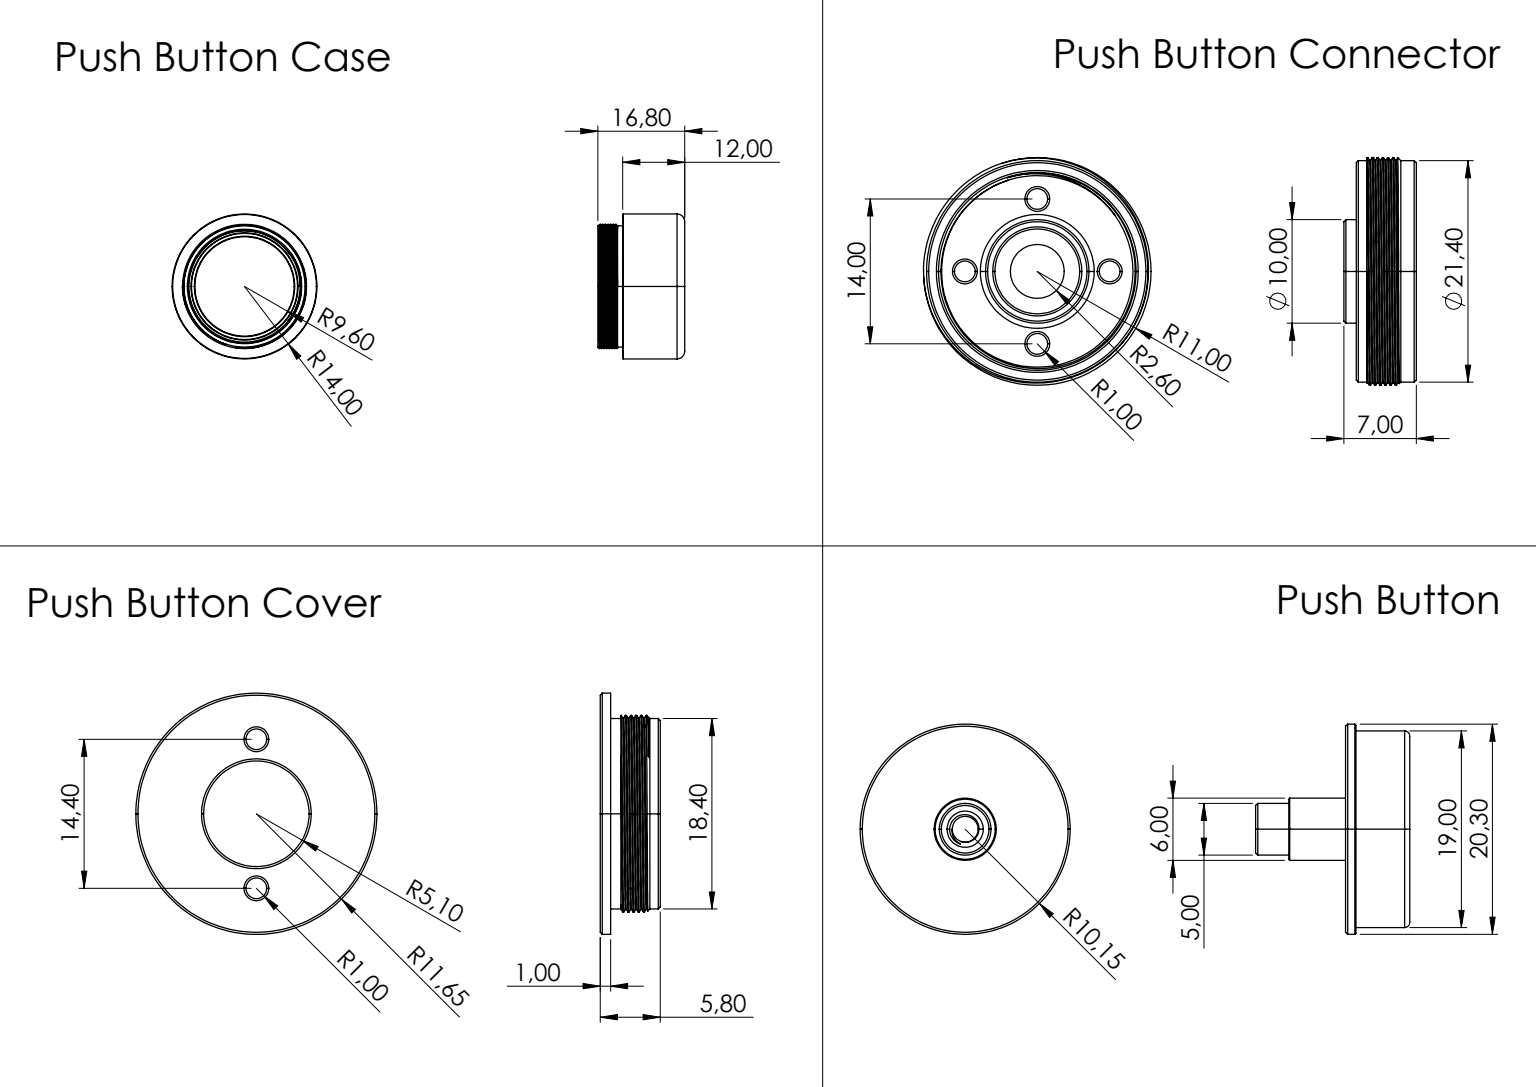
ISO-10303-21;
HEADER;
FILE_DESCRIPTION (('STEP AP214'),
    '1' );
FILE_NAME ('Push Button Cover.step',
    '2026-10-07T19:06:49',
    ( '' ),
    ( '' ),
    'SwSTEP 2.0',
    'SolidWorks 2020',
    '' );
FILE_SCHEMA (( 'AUTOMOTIVE_DESIGN' ));
ENDSEC;

DATA;
#2=CARTESIAN_POINT ( 'NONE',  ( 2.783482194004999855, -79.54451332859899537, 9.108908728793998932 ) ) ;
#10=ORIENTED_EDGE ( 'NONE', *, *, #20290, .T. ) ;
#20=CARTESIAN_POINT ( 'NONE',  ( 4.897371265365999982, -76.96065194988499059, 7.847181321287999722 ) ) ;
#42=CARTESIAN_POINT ( 'NONE',  ( -6.243826001791999758, -76.87571332859899087, 7.064314876436000645 ) ) ;
#56=CARTESIAN_POINT ( 'NONE',  ( 1.899930039692999895, -78.36919415034600434, 9.535935523283001203 ) ) ;
#70=FACE_OUTER_BOUND ( 'NONE', #58213, .T. ) ;
#83=AXIS2_PLACEMENT_3D ( 'NONE', #16611, #21316, #34596 ) ;
#85=CARTESIAN_POINT ( 'NONE',  ( -11.65000000000000036, -75.20000000000000284, 0.000000000000000000 ) ) ;
#89=VERTEX_POINT ( 'NONE', #22267 ) ;
#93=CARTESIAN_POINT ( 'NONE',  ( 3.039902587998999817, -77.28013998579800159, -9.045419714114000698 ) ) ;
#100=CARTESIAN_POINT ( 'NONE',  ( -9.706274203897999442, -78.20406332859900544, -1.344096209030999800 ) ) ;
#101=FACE_OUTER_BOUND ( 'NONE', #29091, .T. ) ;
#107=B_SPLINE_CURVE_WITH_KNOTS ( 'NONE', 3,
 ( #7548, #48867, #4281, #31114, #3130, #21981 ),
 .UNSPECIFIED., .F., .F.,
 ( 4, 2, 4 ),
 ( 0.000000000000000000, 0.5000000000000000000, 1.000000000000000000 ),
 .UNSPECIFIED. ) ;
#109=CARTESIAN_POINT ( 'NONE',  ( 1.243547092045969915, -77.53541666666666288, -9.500000000000000000 ) ) ;
#111=CARTESIAN_POINT ( 'NONE',  ( -5.219189444926520594, -79.47847823290939573, -7.938071756665344481 ) ) ;
#112=DIRECTION ( 'NONE',  ( 0.000000000000000000, 0.7071067811866525998, -0.7071067811864425456 ) ) ;
#113=CARTESIAN_POINT ( 'NONE',  ( -5.761654615528584600, -79.37404003602567570, -7.593432905074549488 ) ) ;
#124=CARTESIAN_POINT ( 'NONE',  ( 0.000000000000000000, -75.00000000000000000, -7.200000000000000178 ) ) ;
#131=CARTESIAN_POINT ( 'NONE',  ( 8.300970689365456678, -78.50833333333332575, -4.784380313523530326 ) ) ;
#138=CARTESIAN_POINT ( 'NONE',  ( 2.459440699436000077, -77.29584903538302854, -9.171074077620000153 ) ) ;
#141=CARTESIAN_POINT ( 'NONE',  ( -9.499999999999998224, -77.31041666666664014, -1.243547092045960367 ) ) ;
#182=CARTESIAN_POINT ( 'NONE',  ( -9.065329452404249366, -79.37552650030312407, 2.840436040226053560 ) ) ;
#198=AXIS2_PLACEMENT_3D ( 'NONE', #57985, #8985, #18719 ) ;
#217=CARTESIAN_POINT ( 'NONE',  ( 8.824144518603999288, -79.29006001420199823, -3.570895061352000077 ) ) ;
#227=FACE_OUTER_BOUND ( 'NONE', #43271, .T. ) ;
#233=VERTEX_POINT ( 'NONE', #25182 ) ;
#261=CARTESIAN_POINT ( 'NONE',  ( -7.282392150664000141, -77.69888667140099869, 6.502067388700999651 ) ) ;
#294=CARTESIAN_POINT ( 'NONE',  ( 8.002843206562666012, -78.09666666666663559, 5.305121725754472273 ) ) ;
#311=AXIS2_PLACEMENT_3D ( 'NONE', #35658, #30929, #8510 ) ;
#318=CARTESIAN_POINT ( 'NONE',  ( 7.430757984336000099, -77.37342305011499377, 5.911115298933000695 ) ) ;
#336=CARTESIAN_POINT ( 'NONE',  ( 8.828604248290998768, -77.09468998579799859, -4.107095029376999662 ) ) ;
#343=CARTESIAN_POINT ( 'NONE',  ( -9.500000000000000000, -77.79999999999999716, 0.000000000000000000 ) ) ;
#346=CARTESIAN_POINT ( 'NONE',  ( 8.913108430814103755, -77.00000000000000000, -3.200251741501357383 ) ) ;
#347=LINE ( 'NONE', #54049, #11944 ) ;
#348=CARTESIAN_POINT ( 'NONE',  ( 1.899930039692999895, -78.42929805011500832, 9.535935523283001203 ) ) ;
#359=DIRECTION ( 'NONE',  ( 0.000000000000000000, 1.000000000000000000, 0.000000000000000000 ) ) ;
#373=DIRECTION ( 'NONE',  ( 1.000000000000000000, 0.000000000000000000, 0.000000000000000000 ) ) ;
#376=( LENGTH_UNIT ( ) NAMED_UNIT ( * ) SI_UNIT ( .MILLI., .METRE. ) );
#389=CARTESIAN_POINT ( 'NONE',  ( -3.218338554480999925, -78.22738998579799841, -9.136931980783000284 ) ) ;
#395=EDGE_LOOP ( 'NONE', ( #41385, #43194, #13742, #37838 ) ) ;
#401=CARTESIAN_POINT ( 'NONE',  ( -8.419758540101616617, -79.43829028770473144, -4.400681399932081739 ) ) ;
#428=CARTESIAN_POINT ( 'NONE',  ( 0.7635722663974530144, -77.01859038055819440, 9.343284614800793975 ) ) ;
#503=CARTESIAN_POINT ( 'NONE',  ( -8.717770243732999802, -79.47198667140099815, 4.088898379276000306 ) ) ;
#504=DIRECTION ( 'NONE',  ( 0.000000000000000000, 1.000000000000000000, 0.000000000000000000 ) ) ;
#535=ORIENTED_EDGE ( 'NONE', *, *, #50020, .F. ) ;
#536=DIRECTION ( 'NONE',  ( 0.000000000000000000, 0.7071067811866525998, -0.7071067811864425456 ) ) ;
#549=CARTESIAN_POINT ( 'NONE',  ( -6.920864301812000186, -77.01268501420199186, 6.182201926393999791 ) ) ;
#601=ADVANCED_FACE ( 'NONE', ( #35967 ), #30933, .T. ) ;
#609=CARTESIAN_POINT ( 'NONE',  ( 8.256620083228000340, -77.33895194988498645, -4.688888258373000717 ) ) ;
#627=CARTESIAN_POINT ( 'NONE',  ( 9.014599915542000019, -77.66018998579799870, 3.680982378367999797 ) ) ;
#630=MECHANICAL_DESIGN_GEOMETRIC_PRESENTATION_REPRESENTATION('',(#12843),#25113);
#636=CARTESIAN_POINT ( 'NONE',  ( 9.443547551318811628, -77.00000000000000000, 0.1845321678459553028 ) ) ;
#643=CARTESIAN_POINT ( 'NONE',  ( 6.099999999940000528, -80.79999999975800051, 5.338249915816000005E-09 ) ) ;
#674=ORIENTED_EDGE ( 'NONE', *, *, #44519, .F. ) ;
#705=FACE_OUTER_BOUND ( 'NONE', #29095, .T. ) ;
#742=ORIENTED_EDGE ( 'NONE', *, *, #42939, .F. ) ;
#752=CARTESIAN_POINT ( 'NONE',  ( -3.329695900066999670, -78.41871001420200571, -9.453077866293002174 ) ) ;
#759=DIRECTION ( 'NONE',  ( 0.000000000000000000, 0.000000000000000000, -1.000000000000000000 ) ) ;
#773=CARTESIAN_POINT ( 'NONE',  ( -5.809342935555999787, -78.93238667140099096, 7.891128111295000025 ) ) ;
#806=CARTESIAN_POINT ( 'NONE',  ( 9.468750000004000356, -79.53124999999600675, -6.681056941828999630E-10 ) ) ;
#821=EDGE_CURVE ( 'NONE', #25723, #3607, #50108, .T. ) ;
#839=CARTESIAN_POINT ( 'NONE',  ( -8.920186055527000946, -77.16191332859899887, 3.688297430249000364 ) ) ;
#845=FACE_OUTER_BOUND ( 'NONE', #7013, .T. ) ;
#866=CARTESIAN_POINT ( 'NONE',  ( 0.9783655976132111798, -77.00000000000000000, 9.249733681752722703 ) ) ;
#869=CARTESIAN_POINT ( 'NONE',  ( 9.235752227612000098, -79.39493998579798983, 1.834089355993999915 ) ) ;
#887=EDGE_CURVE ( 'NONE', #29780, #37236, #38592, .T. ) ;
#892=CARTESIAN_POINT ( 'NONE',  ( 1.009320482739999969, -77.49657694988499657, 9.441330439200999791 ) ) ;
#901=CARTESIAN_POINT ( 'NONE',  ( -8.300970689365472666, -77.75833333333333997, 4.784380313523514339 ) ) ;
#956=CARTESIAN_POINT ( 'NONE',  ( 1.958352037450999727, -78.23868998579800405, 9.829161269560000136 ) ) ;
#1007=CARTESIAN_POINT ( 'NONE',  ( 7.056385154380720337, -79.75000000000000000, -6.024759004142000940 ) ) ;
#1024=CARTESIAN_POINT ( 'NONE',  ( 9.252740428349003565, -78.02916666666668277, -2.486604901413146607 ) ) ;
#1039=CARTESIAN_POINT ( 'NONE',  ( -0.5475862000146000108, -78.94131001420200278, -10.00738244094000073 ) ) ;
#1054=CARTESIAN_POINT ( 'NONE',  ( -9.221371799403371483, -77.06727193750342053, -2.052095926117649682 ) ) ;
#1057=CARTESIAN_POINT ( 'NONE',  ( -7.459109567305000077, -79.06303667140099378, -6.354485205484000865 ) ) ;
#1075=CARTESIAN_POINT ( 'NONE',  ( -8.895437731725001740, -79.41463998579799011, -4.226908468493999038 ) ) ;
#1091=AXIS2_PLACEMENT_3D ( 'NONE', #18206, #13750, #55665 ) ;
#1119=CARTESIAN_POINT ( 'NONE',  ( 9.515085579998999066, -77.75946167140099874, 0.3080020932329999850 ) ) ;
#1130=CARTESIAN_POINT ( 'NONE',  ( 6.100000000000000533, -80.79999999999999716, 0.000000000000000000 ) ) ;
#1134=EDGE_CURVE ( 'NONE', #37723, #31238, #6712, .T. ) ;
#1136=CARTESIAN_POINT ( 'NONE',  ( 4.009386773507102042, -79.41013248972129190, -8.520383303337226266 ) ) ;
#1158=CARTESIAN_POINT ( 'NONE',  ( 6.052764987364000149, -79.37291332859899740, -7.354162135516000731 ) ) ;
#1177=CARTESIAN_POINT ( 'NONE',  ( -9.204193785523999694, -77.14980194988498852, -2.332437886131999871 ) ) ;
#1204=CYLINDRICAL_SURFACE ( 'NONE', #30513, 9.500000000000000000 ) ;
#1213=CIRCLE ( 'NONE', #8729, 9.499999999999996447 ) ;
#1230=B_SPLINE_CURVE_WITH_KNOTS ( 'NONE', 3,
 ( #22828, #141, #18409, #57669, #53244, #53839, #17225, #26948, #36401, #54129, #35214, #44981, #40248, #35809, #35510, #13670, #31666, #12793 ),
 .UNSPECIFIED., .F., .F.,
 ( 4, 2, 2, 2, 2, 2, 2, 2, 4 ),
 ( 0.000000000000000000, 0.1250000000000000833, 0.2500000000000001665, 0.3750000000000002220, 0.5000000000000002220, 0.6250000000000002220, 0.7500000000000001110, 0.8750000000000001110, 1.000000000000000000 ),
 .UNSPECIFIED. ) ;
#1240=CARTESIAN_POINT ( 'NONE',  ( 6.874531804813999614, -78.06448998579800502, -7.293035489291000317 ) ) ;
#1246=CARTESIAN_POINT ( 'NONE',  ( -8.428125188755409170, -79.36138179854771124, 4.406741964346048590 ) ) ;
#1258=CARTESIAN_POINT ( 'NONE',  ( 9.500000000000000000, -79.14999999999999147, 0.000000000000000000 ) ) ;
#1283=CARTESIAN_POINT ( 'NONE',  ( 7.479653633103032995, -77.95140769025543648, 5.651087642253929566 ) ) ;
#1299=CARTESIAN_POINT ( 'NONE',  ( -1.000000000000000000, -78.00000000000000000, 7.200000000000000178 ) ) ;
#1304=CARTESIAN_POINT ( 'NONE',  ( 8.300970689365456678, -78.00833333333332575, -4.784380313523530326 ) ) ;
#1306=EDGE_CURVE ( 'NONE', #10320, #25686, #34712, .T. ) ;
#1317=VERTEX_POINT ( 'NONE', #7865 ) ;
#1326=ORIENTED_EDGE ( 'NONE', *, *, #45707, .F. ) ;
#1338=CARTESIAN_POINT ( 'NONE',  ( -8.932802644879007659, -77.57622193750340500, -3.074066805765899080 ) ) ;
#1366=CARTESIAN_POINT ( 'NONE',  ( 7.507056363060000237, -79.76904805011500343, -5.572808305725000189 ) ) ;
#1370=CARTESIAN_POINT ( 'NONE',  ( 9.252740428348992907, -77.17083333333333428, 2.486604901413179025 ) ) ;
#1386=ADVANCED_FACE ( 'NONE', ( #41198 ), #6893, .F. ) ;
#1416=CARTESIAN_POINT ( 'NONE',  ( -2.226051307435857662, -77.00624999999999432, -9.265603215652616242 ) ) ;
#1422=SHAPE_REPRESENTATION ( 'Push Button Cover', ( #43526 ), #24646 ) ;
#1426=CARTESIAN_POINT ( 'NONE',  ( -0.5312504855272001114, -78.63049415034599576, -9.708839960653000034 ) ) ;
#1499=EDGE_LOOP ( 'NONE', ( #5788, #41984, #28707, #17470, #27775, #26159 ) ) ;
#1517=CARTESIAN_POINT ( 'NONE',  ( -9.155305986995932344, -76.99999999999998579, 1.687095892431314637 ) ) ;
#1527=EDGE_CURVE ( 'NONE', #5139, #52771, #40497, .T. ) ;
#1531=CARTESIAN_POINT ( 'NONE',  ( -8.093517052318336624, -79.35576814611899010, 4.979337055998752426 ) ) ;
#1540=ORIENTED_EDGE ( 'NONE', *, *, #15656, .T. ) ;
#1568=CYLINDRICAL_SURFACE ( 'NONE', #18933, 1.000000000000000000 ) ;
#1581=AXIS2_PLACEMENT_3D ( 'NONE', #4302, #35280, #26150 ) ;
#1584=AXIS2_PLACEMENT_3D ( 'NONE', #55642, #9900, #14892 ) ;
#1608=CARTESIAN_POINT ( 'NONE',  ( 7.265173101945999967, -78.12837668086899612, 6.414655419558000560 ) ) ;
#1631=CARTESIAN_POINT ( 'NONE',  ( -9.595602112029999020, -78.08161001420199909, -1.328770664336999863 ) ) ;
#1639=CARTESIAN_POINT ( 'NONE',  ( 0.000000000000000000, -80.79999999999999716, -9.000000000000000000 ) ) ;
#1650=CARTESIAN_POINT ( 'NONE',  ( 1.848914204786999971, -79.30291332859900422, 9.561723555723999013 ) ) ;
#1652=CARTESIAN_POINT ( 'NONE',  ( 0.000000000000000000, -79.79999999999999716, -9.199999999999999289 ) ) ;
#1659=CARTESIAN_POINT ( 'NONE',  ( -6.090475762158000350, -79.49994805011499466, 7.362120511650999788 ) ) ;
#1679=CARTESIAN_POINT ( 'NONE',  ( 7.689480989199970473, -79.19964970209089472, 5.578385363880753012 ) ) ;
#1686=DIRECTION ( 'NONE',  ( 0.000000000000000000, 1.000000000000000000, 0.000000000000000000 ) ) ;
#1695=CARTESIAN_POINT ( 'NONE',  ( 8.533343070146999665, -77.28601001420200589, -3.969738581741999450 ) ) ;
#1700=CARTESIAN_POINT ( 'NONE',  ( 6.799660072434999591, -77.38031332859900147, -6.851122554325000280 ) ) ;
#1713=CARTESIAN_POINT ( 'NONE',  ( -3.039602602086000083, -79.10954415034599663, -9.236151215514999180 ) ) ;
#1738=ORIENTED_EDGE ( 'NONE', *, *, #53660, .F. ) ;
#1740=EDGE_CURVE ( 'NONE', #34146, #1317, #10335, .T. ) ;
#1746=ORIENTED_EDGE ( 'NONE', *, *, #40301, .T. ) ;
#1747=VERTEX_POINT ( 'NONE', #53544 ) ;
#1750=CARTESIAN_POINT ( 'NONE',  ( 8.582508435409000214, -76.84333998579799641, -4.171307237795000233 ) ) ;
#1762=CARTESIAN_POINT ( 'NONE',  ( 1.900228162289573586, -78.40847913613843900, 9.537431829883434631 ) ) ;
#1805=ADVANCED_BREP_SHAPE_REPRESENTATION ( '', ( #17895, #43526 ), #24646 ) ;
#1811=CARTESIAN_POINT ( 'NONE',  ( -7.401644128749154561, -77.00000000000002842, -5.852483073979606765 ) ) ;
#1825=AXIS2_PLACEMENT_3D ( 'NONE', #48424, #20395, #7104 ) ;
#1834=ORIENTED_EDGE ( 'NONE', *, *, #5380, .F. ) ;
#1858=CARTESIAN_POINT ( 'NONE',  ( -8.997179024602999675, -79.15920584965400053, 3.687079342327000298 ) ) ;
#1906=CARTESIAN_POINT ( 'NONE',  ( -5.674993058560000136, -78.89776001420199236, -8.260872093916999503 ) ) ;
#1911=VERTEX_POINT ( 'NONE', #57674 ) ;
#1918=CARTESIAN_POINT ( 'NONE',  ( 0.000000000000000000, -76.00000000000000000, 0.000000000000000000 ) ) ;
#1927=CARTESIAN_POINT ( 'NONE',  ( -0.5292728922702000238, -78.69131001420200278, -9.672698560386999489 ) ) ;
#1946=CARTESIAN_POINT ( 'NONE',  ( -6.239533324134999503, -79.44973998579799002, -7.619964241536999694 ) ) ;
#1952=CARTESIAN_POINT ( 'NONE',  ( 9.377128579935000374, -78.37869514476064126, -2.571625947824999869 ) ) ;
#1957=CARTESIAN_POINT ( 'NONE',  ( -2.317989000404999889, -79.73555194988499295, -9.269382932261999386 ) ) ;
#1968=B_SPLINE_CURVE_WITH_KNOTS ( 'NONE', 3,
 ( #13129, #31125, #31425, #49162, #26706, #40305, #58313, #17875, #23747, #14300, #10472, #28750, #1338, #41761, #15182, #28458, #46506, #6032, #46800, #32588, #5168, #41176, #10772, #24041, #32293, #28162, #33174, #36739, #37615, #55339, #1054, #27584, #5740, #54757, #42056 ),
 .UNSPECIFIED., .F., .F.,
 ( 4, 1, 1, 1, 1, 1, 1, 1, 1, 1, 1, 1, 1, 1, 1, 1, 1, 1, 1, 1, 1, 1, 1, 1, 1, 1, 1, 1, 1, 1, 1, 1, 4 ),
 ( 0.000000000000000000, 0.01250064086135114876, 0.04500059900521829331, 0.07750055714907158610, 0.1100005152929402902, 0.1425004734368089665, 0.1750004315807084654, 0.2075003897244847573, 0.2400003478684150648, 0.2725003060121913845, 0.3050002641561216365, 0.3375002223000519441, 0.3700001804438282638, 0.4025001385877585158, 0.4350000967315347800, 0.4675000548754650875, 0.5000000130192413517, 0.5324999711631716037, 0.5649999293071019668, 0.5974998874508783420, 0.6299998455948085940, 0.6624998037385848582, 0.6949997618825151102, 0.7274997200262914854, 0.7599996781702217374, 0.7924996363141521005, 0.8249995944579283647, 0.8574995526018586167, 0.8899995107456349919, 0.9224994688895652439, 0.9549994270333415081, 0.9874993851772717601, 1.000000000000000000 ),
 .UNSPECIFIED. ) ;
#1976=CARTESIAN_POINT ( 'NONE',  ( 8.331125690395985828, -79.18975047827684932, 4.575408606511675913 ) ) ;
#1991=ADVANCED_FACE ( 'NONE', ( #46760 ), #55002, .T. ) ;
#1992=DIRECTION ( 'NONE',  ( 0.000000000000000000, -1.000000000000000000, 0.000000000000000000 ) ) ;
#1998=CARTESIAN_POINT ( 'NONE',  ( 2.486604901413132840, -77.15416666666668277, 9.252740428349005342 ) ) ;
#2051=CARTESIAN_POINT ( 'NONE',  ( 9.426477049435000310, -77.25026915034599995, -1.139727483088999849 ) ) ;
#2055=CARTESIAN_POINT ( 'NONE',  ( -9.632966741362359642, -78.06007913613844096, -1.333944807945767863 ) ) ;
#2061=CARTESIAN_POINT ( 'NONE',  ( 1.243547092045969915, -78.03541666666666288, -9.500000000000000000 ) ) ;
#2065=CARTESIAN_POINT ( 'NONE',  ( -9.252740428349007118, -78.87916666666666288, 2.486604901413125734 ) ) ;
#2093=AXIS2_PLACEMENT_3D ( 'NONE', #49507, #50097, #22330 ) ;
#2109=CARTESIAN_POINT ( 'NONE',  ( -9.372585790538636275, -77.88499999999999091, 1.790612804732441221 ) ) ;
#2114=CARTESIAN_POINT ( 'NONE',  ( -9.379567534213441249, -79.38691803057906782, 1.514930929802611681 ) ) ;
#2146=FACE_OUTER_BOUND ( 'NONE', #52697, .T. ) ;
#2164=LINE ( 'NONE', #46757, #39820 ) ;
#2193=CARTESIAN_POINT ( 'NONE',  ( 6.711318802534000483, -78.57268667140098728, 7.292371261484999145 ) ) ;
#2212=CARTESIAN_POINT ( 'NONE',  ( 6.797895215277000247, -78.12826332859900447, -7.211733462747999646 ) ) ;
#2237=CARTESIAN_POINT ( 'NONE',  ( -8.918806285220000518, -78.11739514476064983, 3.872830773119999126 ) ) ;
#2246=CARTESIAN_POINT ( 'NONE',  ( 4.784380313523522332, -77.23333333333332007, 8.300970689365462007 ) ) ;
#2257=CARTESIAN_POINT ( 'NONE',  ( 6.135231488085603146, -79.21900635011196812, 7.253197741126338194 ) ) ;
#2278=CARTESIAN_POINT ( 'NONE',  ( -7.361960514518000487, -77.56153667140098662, -6.036001273387999966 ) ) ;
#2315=EDGE_LOOP ( 'NONE', ( #8172, #22576, #4098, #16468 ) ) ;
#2320=ORIENTED_EDGE ( 'NONE', *, *, #58012, .F. ) ;
#2324=ORIENTED_EDGE ( 'NONE', *, *, #52934, .F. ) ;
#2338=CARTESIAN_POINT ( 'NONE',  ( -5.506559303151407292, -78.62622913613842002, -8.015689466314336542 ) ) ;
#2346=CARTESIAN_POINT ( 'NONE',  ( -9.252740428349001789, -77.92083333333333428, -2.486604901413163926 ) ) ;
#2395=EDGE_LOOP ( 'NONE', ( #43208, #30951, #22703, #57067 ) ) ;
#2438=LINE ( 'NONE', #38724, #47230 ) ;
#2448=CARTESIAN_POINT ( 'NONE',  ( 4.044903269867999640, -79.05999999999998806, -8.595856998426999240 ) ) ;
#2475=CARTESIAN_POINT ( 'NONE',  ( 1.936520525790000002, -78.61623667140099769, 9.719586767747999900 ) ) ;
#2485=CARTESIAN_POINT ( 'NONE',  ( -9.450266643504305009, -79.40799665456589196, -0.9830318362740778637 ) ) ;
#2491=CARTESIAN_POINT ( 'NONE',  ( 8.546298008199000762, -78.65086332859900153, -5.018094164374000243 ) ) ;
#2494=CIRCLE ( 'NONE', #39213, 9.000000000000000000 ) ;
#2521=CARTESIAN_POINT ( 'NONE',  ( 8.384816012895999648, -78.85774514476065633, -4.923277454554000343 ) ) ;
#2542=CARTESIAN_POINT ( 'NONE',  ( 4.369668091130538556, -79.23660998577489067, 8.435227713305813779 ) ) ;
#2547=ORIENTED_EDGE ( 'NONE', *, *, #21590, .T. ) ;
#2550=CONICAL_SURFACE ( 'NONE', #34593, 9.099999999966000175, 0.7853981633972997312 ) ;
#2563=CARTESIAN_POINT ( 'NONE',  ( -5.838193839761721016, -77.22708333333332575, 7.596835002782687418 ) ) ;
#2578=VECTOR ( 'NONE', #112, 1000.000000000000000 ) ;
#2619=CARTESIAN_POINT ( 'NONE',  ( 3.861138328465000047, -76.85095248368000398, 8.493887087553000370 ) ) ;
#2624=CARTESIAN_POINT ( 'NONE',  ( -7.604857126344345630, -78.49557913613843141, 6.061321726079917482 ) ) ;
#2717=CARTESIAN_POINT ( 'NONE',  ( 4.411570631796044140, -76.99999999999998579, 8.157888388493256926 ) ) ;
#2721=CARTESIAN_POINT ( 'NONE',  ( 9.345760913908002010, -78.40230194988500045, 2.683384691900000174 ) ) ;
#2750=VERTEX_POINT ( 'NONE', #3102 ) ;
#2762=CARTESIAN_POINT ( 'NONE',  ( 4.349579488465999511, -79.03151332859899014, 8.780633650160998727 ) ) ;
#2779=CARTESIAN_POINT ( 'NONE',  ( 6.711318802534000483, -78.25891332859899308, 7.292371261484999145 ) ) ;
#2787=CARTESIAN_POINT ( 'NONE',  ( 3.938458446976999205, -79.30999999999998806, -8.369650235310999165 ) ) ;
#2809=CARTESIAN_POINT ( 'NONE',  ( 6.584508673715998128, -78.46579514476064787, 7.154582167228999090 ) ) ;
#2820=VERTEX_POINT ( 'NONE', #8379 ) ;
#2827=CARTESIAN_POINT ( 'NONE',  ( 8.035977331916674515, -79.19462052551928366, 5.075416816263699005 ) ) ;
#2833=CARTESIAN_POINT ( 'NONE',  ( 1.861192509982939169, -79.69030282387936381, -9.372352437101028499 ) ) ;
#2846=CARTESIAN_POINT ( 'NONE',  ( 7.412894021246999365, -77.70291167140099731, -5.973338413043999928 ) ) ;
#2852=CARTESIAN_POINT ( 'NONE',  ( 0.000000000000000000, -79.65000000003199432, 0.000000000000000000 ) ) ;
#2910=CARTESIAN_POINT ( 'NONE',  ( -9.003040227835604981, -79.32727112472369413, -3.132519729896531935 ) ) ;
#2916=CARTESIAN_POINT ( 'NONE',  ( -7.596835002782739821, -78.84791666666669130, 5.838193839761659731 ) ) ;
#2945=CARTESIAN_POINT ( 'NONE',  ( -3.012268937172999816, -79.85615333806700278, -9.005103130722002192 ) ) ;
#2968=CARTESIAN_POINT ( 'NONE',  ( 0.000000000000000000, -74.70999999999999375, 0.000000000000000000 ) ) ;
#3006=CARTESIAN_POINT ( 'NONE',  ( -7.530775182571000315, -78.18455194988499102, -6.150709233331999037 ) ) ;
#3012=VERTEX_POINT ( 'NONE', #46175 ) ;
#3014=DIRECTION ( 'NONE',  ( 0.000000000000000000, -1.000000000000000000, 0.000000000000000000 ) ) ;
#3038=EDGE_CURVE ( 'NONE', #22499, #1747, #34876, .T. ) ;
#3040=FILL_AREA_STYLE_COLOUR ( '', #28459 ) ;
#3047=EDGE_LOOP ( 'NONE', ( #11821, #26978, #6807, #19530, #9731, #11234 ) ) ;
#3051=CARTESIAN_POINT ( 'NONE',  ( -7.459109567305000077, -79.24926332859899958, -6.354485205484000865 ) ) ;
#3067=EDGE_CURVE ( 'NONE', #31891, #15380, #15330, .T. ) ;
#3070=CARTESIAN_POINT ( 'NONE',  ( -9.706274203897999442, -78.01783667140099965, -1.344096209030999800 ) ) ;
#3076=CARTESIAN_POINT ( 'NONE',  ( 4.784380313523556083, -78.96666666666669698, -8.300970689365444244 ) ) ;
#3094=CARTESIAN_POINT ( 'NONE',  ( 0.000000000000000000, -75.00000000000000000, 0.000000000000000000 ) ) ;
#3102=CARTESIAN_POINT ( 'NONE',  ( -11.65000000000000036, -76.00000000000000000, 0.000000000000000000 ) ) ;
#3124=CARTESIAN_POINT ( 'NONE',  ( -3.112989155534594321, -79.30136502081413141, 8.977538257521471721 ) ) ;
#3126=ORIENTED_EDGE ( 'NONE', *, *, #57860, .F. ) ;
#3130=CARTESIAN_POINT ( 'NONE',  ( 7.217860716171294655, -79.49333333333333940, -6.227832364471528770 ) ) ;
#3142=CARTESIAN_POINT ( 'NONE',  ( -9.001945887299001470, -77.53326167140099301, -3.097861235667999757 ) ) ;
#3205=CARTESIAN_POINT ( 'NONE',  ( -9.500350562740681681, -79.30722730559423894, -0.7959580027764865395 ) ) ;
#3206=CARTESIAN_POINT ( 'NONE',  ( 2.486604901413172808, -78.04583333333330586, -9.252740428348992907 ) ) ;
#3239=CARTESIAN_POINT ( 'NONE',  ( 5.875583596582999668, -79.57968667140100649, 7.634009735705999944 ) ) ;
#3259=CARTESIAN_POINT ( 'NONE',  ( -0.7479529023060000892, -77.80888084965400253, -9.465622776916999825 ) ) ;
#3289=LINE ( 'NONE', #43440, #55934 ) ;
#3295=CARTESIAN_POINT ( 'NONE',  ( -3.039602602086000083, -79.16964805011500061, -9.236151215514999180 ) ) ;
#3329=VECTOR ( 'NONE', #58150, 1000.000000000000114 ) ;
#3336=CARTESIAN_POINT ( 'NONE',  ( -7.675809325333999844, -78.31138667140099585, -6.269164879585000349 ) ) ;
#3387=CARTESIAN_POINT ( 'NONE',  ( 9.539544502573999551, -79.32444805011499511, 0.5400218831816999687 ) ) ;
#3394=CARTESIAN_POINT ( 'NONE',  ( 0.000000000000000000, -74.70999999999999375, 0.000000000000000000 ) ) ;
#3404=ORIENTED_EDGE ( 'NONE', *, *, #821, .T. ) ;
#3406=CARTESIAN_POINT ( 'NONE',  ( -1.469979871250949310, -79.28716761129145141, 9.385467292518239191 ) ) ;
#3454=CIRCLE ( 'NONE', #47809, 9.199999999999999289 ) ;
#3482=CARTESIAN_POINT ( 'NONE',  ( -7.898810015907999471, -77.87186001420199943, -5.922837236108999370 ) ) ;
#3507=EDGE_CURVE ( 'NONE', #40288, #25723, #28706, .T. ) ;
#3519=CARTESIAN_POINT ( 'NONE',  ( -5.199237357848000229, -79.90086001420199580, -8.238468209311999857 ) ) ;
#3538=CARTESIAN_POINT ( 'NONE',  ( 1.009320482739999969, -77.55668084965400055, 9.441330439200999791 ) ) ;
#3566=ORIENTED_EDGE ( 'NONE', *, *, #40614, .T. ) ;
#3571=CARTESIAN_POINT ( 'NONE',  ( 3.574993757284770979, -77.00000000000001421, 8.552566962383416183 ) ) ;
#3574=CARTESIAN_POINT ( 'NONE',  ( -5.764562846862999912, -78.99544805011498738, 7.830301022820999712 ) ) ;
#3606=CARTESIAN_POINT ( 'NONE',  ( -1.243547092045951263, -78.51458333333333428, -9.500000000000003553 ) ) ;
#3607=VERTEX_POINT ( 'NONE', #16531 ) ;
#3609=EDGE_LOOP ( 'NONE', ( #5179, #30253, #35549, #13398 ) ) ;
#3613=CARTESIAN_POINT ( 'NONE',  ( -9.565996717342001077, -79.14193998579798972, -1.527434585433000036 ) ) ;
#3618=ORIENTED_EDGE ( 'NONE', *, *, #47736, .F. ) ;
#3625=CARTESIAN_POINT ( 'NONE',  ( -6.673815826044733335, -79.46282625145217082, -6.760806027906673954 ) ) ;
#3641=CARTESIAN_POINT ( 'NONE',  ( -8.300970689365446020, -78.84166666666665435, -4.784380313523547201 ) ) ;
#3669=CARTESIAN_POINT ( 'NONE',  ( -2.317989000404999889, -79.61534415034599022, -9.269382932261999386 ) ) ;
#3687=CARTESIAN_POINT ( 'NONE',  ( 1.484863747559565628, -79.26247634984721913, 9.383218303840022756 ) ) ;
#3751=EDGE_CURVE ( 'NONE', #41331, #18799, #13852, .T. ) ;
#3768=CARTESIAN_POINT ( 'NONE',  ( 9.685708259213999582, -77.51688667140099653, 1.223589504196999966 ) ) ;
#3778=ADVANCED_FACE ( 'NONE', ( #29700 ), #29807, .T. ) ;
#3802=ADVANCED_FACE ( 'NONE', ( #42725 ), #11435, .T. ) ;
#3816=EDGE_CURVE ( 'NONE', #39245, #23213, #25284, .T. ) ;
#3824=CARTESIAN_POINT ( 'NONE',  ( 4.001451577097999923, -78.02955584965400249, 8.339717337904000161 ) ) ;
#3855=LINE ( 'NONE', #4444, #25802 ) ;
#3857=LINE ( 'NONE', #30990, #48551 ) ;
#3860=CARTESIAN_POINT ( 'NONE',  ( 6.584508673715999905, -78.50595584965400064, 7.154582167228999978 ) ) ;
#3866=CARTESIAN_POINT ( 'NONE',  ( 2.951189771924321192, -78.14999999999996305, 9.074256859245705797 ) ) ;
#3875=DIRECTION ( 'NONE',  ( 0.000000000000000000, -1.000000000000000000, 0.000000000000000000 ) ) ;
#3876=ORIENTED_EDGE ( 'NONE', *, *, #16713, .F. ) ;
#3896=CARTESIAN_POINT ( 'NONE',  ( 4.299985066278999568, -78.96773998579799070, 8.680515821880000260 ) ) ;
#3906=CARTESIAN_POINT ( 'NONE',  ( -9.500000000000001776, -77.41041666666667709, -1.243547092045959923 ) ) ;
#3915=CARTESIAN_POINT ( 'NONE',  ( -4.760969735703844741, -79.21703514507530031, 8.244157308523952565 ) ) ;
#3957=EDGE_CURVE ( 'NONE', #34611, #40996, #52472, .T. ) ;
#3973=CARTESIAN_POINT ( 'NONE',  ( -7.560040866215333111, -79.34781027512715923, 5.752875731716930119 ) ) ;
#4004=CARTESIAN_POINT ( 'NONE',  ( -7.941500096889264171, -78.94666666666665833, -5.274086223140034058 ) ) ;
#4023=ORIENTED_EDGE ( 'NONE', *, *, #56145, .T. ) ;
#4054=CARTESIAN_POINT ( 'NONE',  ( 6.922694868096999521, -76.94662000473400099, -6.559930598350000253 ) ) ;
#4061=CARTESIAN_POINT ( 'NONE',  ( -3.948661938011531092, -79.74013365314458213, -8.441925471967053340 ) ) ;
#4082=FACE_BOUND ( 'NONE', #6449, .T. ) ;
#4098=ORIENTED_EDGE ( 'NONE', *, *, #31074, .F. ) ;
#4108=ORIENTED_EDGE ( 'NONE', *, *, #3507, .T. ) ;
#4115=CARTESIAN_POINT ( 'NONE',  ( -7.264520526674999701, -77.74583084965399848, -6.114261184555999762 ) ) ;
#4140=CARTESIAN_POINT ( 'NONE',  ( -9.504662724600999368, -76.89676498579798647, -2.115138623684999608 ) ) ;
#4153=CARTESIAN_POINT ( 'NONE',  ( -5.600962501326000265, -77.99379805011500366, 7.948110234177999445 ) ) ;
#4160=CARTESIAN_POINT ( 'NONE',  ( -8.872994237323279521, -78.27000000000003865, 3.510218210012939100 ) ) ;
#4186=( NAMED_UNIT ( * ) SI_UNIT ( $, .STERADIAN. ) SOLID_ANGLE_UNIT ( ) );
#4190=CARTESIAN_POINT ( 'NONE',  ( -5.838193839761687265, -78.47291666666666288, -7.596835002782715840 ) ) ;
#4191=CARTESIAN_POINT ( 'NONE',  ( 0.6948940501455999064, -77.49853998579800418, 9.517234252032999109 ) ) ;
#4198=CARTESIAN_POINT ( 'NONE',  ( 7.022198843594999573, -77.93705665246400827, 6.200125618097000135 ) ) ;
#4211=CARTESIAN_POINT ( 'NONE',  ( -9.148289698020947824, -79.42135170196439731, -2.562996480311285019 ) ) ;
#4212=CARTESIAN_POINT ( 'NONE',  ( -9.500000000000000000, -74.70999999999999375, 0.000000000000000000 ) ) ;
#4238=CARTESIAN_POINT ( 'NONE',  ( 5.948947503763784894, -77.81911908264200406, 7.191054624583967048 ) ) ;
#4241=B_SPLINE_SURFACE_WITH_KNOTS ( 'NONE', 3, 3, ( 
 ( #33205, #51543, #46831, #24665, #45951, #46244, #6063, #20239, #14626, #42673, #28785, #37651, #15214, #6357, #24374, #19649, #42386, #32618, #11100 ),
 ( #55961, #10212, #15512, #23488, #1957, #37355, #19950, #41501, #50670, #29080, #38232, #56253, #47125, #15803, #50376, #9923, #41794, #28191, #23779 ),
 ( #27905, #1366, #46541, #5482, #14916, #19362, #55371, #32911, #50955, #1659, #10507, #28490, #24073, #42090, #3387, #42967, #39395, #7811, #16677 ),
 ( #52975, #34658, #25812, #34080, #3669, #21669, #43840, #21382, #33792, #7232, #57403, #38524, #48275, #16961, #34943, #29651, #29365, #30522, #20526 ) ),
 .UNSPECIFIED., .F., .F., .F.,
 ( 4, 4 ),
 ( 4, 1, 1, 1, 1, 1, 1, 1, 1, 1, 1, 1, 1, 1, 1, 1, 4 ),
 ( -0.4015584965371999937, 1.401558496537000043 ),
 ( 0.5889552238806000650, 0.6151492537313000275, 0.6413432835821000211, 0.6675373134327999836, 0.6937313432835999771, 0.7199253731343000506, 0.7461194029851000442, 0.7723134328358000067, 0.7985074626866000003, 0.8247014925372999627, 0.8508955223880999563, 0.8770895522388000298, 0.9032835820896000234, 0.9294776119402999859, 0.9556716417910000594, 0.9818656716417999419, 1.008059701493000171 ),
 .UNSPECIFIED. ) ;
#4275=CARTESIAN_POINT ( 'NONE',  ( -5.548822036515788980, -79.32452569715752588, 7.710984173510062156 ) ) ;
#4281=CARTESIAN_POINT ( 'NONE',  ( 5.442299421053111708, -79.47333333333332916, -7.827182525635441479 ) ) ;
#4302=CARTESIAN_POINT ( 'NONE',  ( 0.000000000000000000, -75.20000000000000284, 0.000000000000000000 ) ) ;
#4305=CARTESIAN_POINT ( 'NONE',  ( -6.380391360217929630, -78.96666666666666856, -7.083361869089003449 ) ) ;
#4309=VERTEX_POINT ( 'NONE', #52100 ) ;
#4347=CARTESIAN_POINT ( 'NONE',  ( -8.160216722324735272, -79.66145833332932114, 4.702279492088285551 ) ) ;
#4356=CARTESIAN_POINT ( 'NONE',  ( -6.446975197297999394, -77.18928667140100686, 7.331209084132000342 ) ) ;
#4360=B_SPLINE_CURVE_WITH_KNOTS ( 'NONE', 3,
 ( #51971, #20663, #23923, #47560, #11528, #7085 ),
 .UNSPECIFIED., .F., .F.,
 ( 4, 2, 4 ),
 ( 0.000000000000000000, 0.5000000000000000000, 1.000000000000000000 ),
 .UNSPECIFIED. ) ;
#4365=CARTESIAN_POINT ( 'NONE',  ( -2.364557222828000072, -79.54490095943376105, 9.257622954664000758 ) ) ;
#4395=CARTESIAN_POINT ( 'NONE',  ( -2.978309893851999846, -79.79237999526598912, -8.903583414616999647 ) ) ;
#4413=CARTESIAN_POINT ( 'NONE',  ( 4.574312611392000072, -77.52515584965399853, 8.320643751074999983 ) ) ;
#4435=CARTESIAN_POINT ( 'NONE',  ( -8.084017119143000585, -76.98881332859899373, -5.230585977929000485 ) ) ;
#4444=CARTESIAN_POINT ( 'NONE',  ( -6.099999999940000528, -80.79999999975800051, -5.338250164827000611E-09 ) ) ;
#4445=CARTESIAN_POINT ( 'NONE',  ( 8.185698792048100358, -77.00000000000001421, 4.534146512987735633 ) ) ;
#4448=CARTESIAN_POINT ( 'NONE',  ( 6.584508673715999905, -78.38574805011499791, 7.154582167228999978 ) ) ;
#4455=CARTESIAN_POINT ( 'NONE',  ( -3.234762833941021931, -78.20250000000001478, 8.977080150340221110 ) ) ;
#4488=CARTESIAN_POINT ( 'NONE',  ( 9.022242495772999860, -77.35293998579798824, -3.108016392540000172 ) ) ;
#4496=CARTESIAN_POINT ( 'NONE',  ( 2.006136628026000235, -78.27093998579799461, -9.477164255927000625 ) ) ;
#4499=CARTESIAN_POINT ( 'NONE',  ( 4.790152371929814912, -79.21780269203372882, -7.968054111795736638 ) ) ;
#4506=CARTESIAN_POINT ( 'NONE',  ( -6.849002874435582200, -79.46067733726329152, -6.583439657378555410 ) ) ;
#4508=CARTESIAN_POINT ( 'NONE',  ( -0.6023433875411666749, -79.42080894732758622, -9.578712713088513908 ) ) ;
#4526=CARTESIAN_POINT ( 'NONE',  ( -8.300970689365446020, -78.34166666666668277, -4.784380313523547201 ) ) ;
#4533=CARTESIAN_POINT ( 'NONE',  ( 9.136202122873999798, -77.42194903538302242, 2.585973524421999237 ) ) ;
#4567=LINE ( 'NONE', #26395, #28221 ) ;
#4573=CARTESIAN_POINT ( 'NONE',  ( -7.688125331226709491, -79.34962435731765140, 5.580139227232765009 ) ) ;
#4592=CARTESIAN_POINT ( 'NONE',  ( -2.684723000728000297, -77.10913667140100358, -9.133676008435999805 ) ) ;
#4611=CARTESIAN_POINT ( 'NONE',  ( 9.504033308897000154, -79.32516001420199814, 0.5380116381770999601 ) ) ;
#4617=CARTESIAN_POINT ( 'NONE',  ( 3.350444873057258022, -79.30441504825350307, -8.644740048361368778 ) ) ;
#4661=CARTESIAN_POINT ( 'NONE',  ( -5.497893974011999418, -77.39866001420199382, -8.200266008636999615 ) ) ;
#4668=CARTESIAN_POINT ( 'NONE',  ( -6.188001695094492050, -79.71856730628915955, -7.220675648484128573 ) ) ;
#4685=PLANE ( 'NONE',  #14153 ) ;
#4696=CARTESIAN_POINT ( 'NONE',  ( -5.083316206963999662, -79.77331332859898794, -8.054784978366999582 ) ) ;
#4715=CARTESIAN_POINT ( 'NONE',  ( 9.475051992780000987, -77.81477305011499368, -0.6170397550469999270 ) ) ;
#4732=DIRECTION ( 'NONE',  ( 0.000000000000000000, 1.000000000000000000, 0.000000000000000000 ) ) ;
#4734=CARTESIAN_POINT ( 'NONE',  ( -4.454645851891000596, -77.35638832859899594, 8.536186251725998986 ) ) ;
#4742=CARTESIAN_POINT ( 'NONE',  ( 8.534835205664490942, -77.00000000000000000, 3.862497297122138296 ) ) ;
#4776=CARTESIAN_POINT ( 'NONE',  ( -2.486604901413153268, -78.50416666666667709, -9.252740428348998236 ) ) ;
#4784=CARTESIAN_POINT ( 'NONE',  ( 9.685875573750999834, -78.88063998579799829, 0.1582452683012000039 ) ) ;
#4799=CARTESIAN_POINT ( 'NONE',  ( -9.380299113924060350, -79.41227555779782676, -1.501938252706041643 ) ) ;
#4801=CARTESIAN_POINT ( 'NONE',  ( 0.000000000000000000, -77.00000000000000000, 0.000000000000000000 ) ) ;
#4815=PRODUCT_DEFINITION ( 'UNKNOWN', '', #22577, #7968 ) ;
#4825=CARTESIAN_POINT ( 'NONE',  ( 7.430757984335999211, -77.45347403538301023, 5.911115298933000695 ) ) ;
#4852=CARTESIAN_POINT ( 'NONE',  ( -5.100000000000000533, -76.79999999999999716, 0.000000000000000000 ) ) ;
#4859=CIRCLE ( 'NONE', #35929, 1.000000000000000000 ) ;
#4943=CARTESIAN_POINT ( 'NONE',  ( -1.179576631548999943, -77.45566001420199598, 9.337310497832001843 ) ) ;
#4964=ORIENTED_EDGE ( 'NONE', *, *, #37684, .T. ) ;
#4980=CARTESIAN_POINT ( 'NONE',  ( -3.858678039026999684, -79.53793998579800473, 8.589155328362998887 ) ) ;
#5002=CARTESIAN_POINT ( 'NONE',  ( 2.459440699436000077, -77.21579805011499786, -9.171074077620000153 ) ) ;
#5003=FACE_OUTER_BOUND ( 'NONE', #38346, .T. ) ;
#5013=CONICAL_SURFACE ( 'NONE', #36113, 1.099999997157999232, 0.7853981633972997312 ) ;
#5020=CARTESIAN_POINT ( 'NONE',  ( 4.982928723802999116, -77.54708998579799584, -8.365578579050000130 ) ) ;
#5032=CARTESIAN_POINT ( 'NONE',  ( -8.997179024602999675, -78.97889415034599381, 3.687079342327000298 ) ) ;
#5056=B_SPLINE_CURVE_WITH_KNOTS ( 'NONE', 3,
 ( #28202, #35965, #22688, #294, #54287, #31823 ),
 .UNSPECIFIED., .F., .F.,
 ( 4, 2, 4 ),
 ( 0.000000000000000000, 0.4999999999999998890, 1.000000000000000000 ),
 .UNSPECIFIED. ) ;
#5060=CARTESIAN_POINT ( 'NONE',  ( -8.314650709467036549, -77.00000000000000000, -4.397163425340465892 ) ) ;
#5116=CIRCLE ( 'NONE', #39063, 9.000000000000000000 ) ;
#5118=CARTESIAN_POINT ( 'NONE',  ( -2.205007487985999770, -77.04364903538302656, 9.235565851336001941 ) ) ;
#5139=VERTEX_POINT ( 'NONE', #49750 ) ;
#5168=CARTESIAN_POINT ( 'NONE',  ( 7.630512808711405803, -77.35002193750341348, 5.569571266600500614 ) ) ;
#5172=CARTESIAN_POINT ( 'NONE',  ( 7.890654042133999901, -77.86386001420198966, 4.760698198672999482 ) ) ;
#5179=ORIENTED_EDGE ( 'NONE', *, *, #6097, .F. ) ;
#5209=DIRECTION ( 'NONE',  ( 0.000000000000000000, -1.000000000000000000, 0.000000000000000000 ) ) ;
#5213=ORIENTED_EDGE ( 'NONE', *, *, #56640, .F. ) ;
#5219=CARTESIAN_POINT ( 'NONE',  ( 9.319018100775748437, -79.16524970259979455, 1.846458293751403135 ) ) ;
#5234=CARTESIAN_POINT ( 'NONE',  ( 8.924962326551000302, -77.79496001420199036, -2.986943611218999983 ) ) ;
#5239=CARTESIAN_POINT ( 'NONE',  ( -9.632028597164000061, -77.19831332859899931, -0.6303035207593999933 ) ) ;
#5268=CARTESIAN_POINT ( 'NONE',  ( -3.778637972659712574, -77.00000000000000000, 8.499186437672962668 ) ) ;
#5280=EDGE_LOOP ( 'NONE', ( #16907, #43622, #39884 ) ) ;
#5285=ORIENTED_EDGE ( 'NONE', *, *, #47801, .F. ) ;
#5290=CARTESIAN_POINT ( 'NONE',  ( -9.391369684923001060, -77.11827694988500070, 1.399863080762999923 ) ) ;
#5321=CARTESIAN_POINT ( 'NONE',  ( 7.685661446562000343, -77.00000000000000000, -5.583959896779000509 ) ) ;
#5332=CARTESIAN_POINT ( 'NONE',  ( 0.000000000000000000, -80.59999999999999432, 0.000000000000000000 ) ) ;
#5344=CARTESIAN_POINT ( 'NONE',  ( -8.944216015804251185, -77.00000000000000000, -2.811381416889873197 ) ) ;
#5351=CARTESIAN_POINT ( 'NONE',  ( -9.307291666739137881, -79.69270833332970483, -0.9752027189503162941 ) ) ;
#5355=CARTESIAN_POINT ( 'NONE',  ( -5.610847844242282001, -77.82499999999998863, 7.718163323371708628 ) ) ;
#5380=EDGE_CURVE ( 'NONE', #36499, #34323, #14580, .T. ) ;
#5406=CARTESIAN_POINT ( 'NONE',  ( 6.559824298179475655, -79.75000000000000000, -6.561935513396097264 ) ) ;
#5433=CARTESIAN_POINT ( 'NONE',  ( -0.8742025125545000996, -79.20261001420199420, 9.984153739810000872 ) ) ;
#5458=CARTESIAN_POINT ( 'NONE',  ( 8.449950666592000559, -78.71463667140099574, -4.961522297560000183 ) ) ;
#5473=CARTESIAN_POINT ( 'NONE',  ( 5.818877114584999788, -79.20403998579800486, 7.945831408065000545 ) ) ;
#5482=CARTESIAN_POINT ( 'NONE',  ( 1.861092857305999937, -79.71054805011500832, -9.371850619045000386 ) ) ;
#5517=ADVANCED_FACE ( 'NONE', ( #52071 ), #43580, .T. ) ;
#5521=CARTESIAN_POINT ( 'NONE',  ( 9.576515689347999682, -77.45311332859900233, 1.209795274715000257 ) ) ;
#5524=CARTESIAN_POINT ( 'NONE',  ( 9.500000000000005329, -77.14374999999998295, -0.7461282552275557700 ) ) ;
#5549=EDGE_LOOP ( 'NONE', ( #7465, #28790, #49499, #535, #12184, #37449, #17548, #17218, #35107 ) ) ;
#5553=CARTESIAN_POINT ( 'NONE',  ( 4.024324870012000233, -79.29007331913099677, -8.363631784355000320 ) ) ;
#5573=CARTESIAN_POINT ( 'NONE',  ( -7.591316436381999821, -77.18132694988500475, -5.703451837412999659 ) ) ;
#5574=PLANE ( 'NONE',  #42337 ) ;
#5638=CARTESIAN_POINT ( 'NONE',  ( -2.370458031814262068, -77.79499999999998749, 9.242975026304343089 ) ) ;
#5665=CARTESIAN_POINT ( 'NONE',  ( 9.500517569907307447, -79.06045223105810749, 1.242907163946308069 ) ) ;
#5685=CARTESIAN_POINT ( 'NONE',  ( 9.426477049435000310, -77.39042403538302040, -1.139727483088999849 ) ) ;
#5705=CARTESIAN_POINT ( 'NONE',  ( 2.486604901413172364, -77.94583333333333997, -9.252740428348998236 ) ) ;
#5740=CARTESIAN_POINT ( 'NONE',  ( -8.539484132404522754, -77.01652175453601501, 3.808411293863636971 ) ) ;
#5776=CARTESIAN_POINT ( 'NONE',  ( -5.838193839761721016, -77.32708333333333428, 7.596835002782687418 ) ) ;
#5787=ORIENTED_EDGE ( 'NONE', *, *, #54972, .T. ) ;
#5788=ORIENTED_EDGE ( 'NONE', *, *, #29018, .F. ) ;
#5797=DIRECTION ( 'NONE',  ( -1.000000000000000000, 0.000000000000000000, 0.000000000000000000 ) ) ;
#5807=CARTESIAN_POINT ( 'NONE',  ( -4.354206273205999622, -77.48393501420198959, 8.343719559825000687 ) ) ;
#5808=CARTESIAN_POINT ( 'NONE',  ( 0.000000000000000000, -79.65000000003199432, 0.000000000000000000 ) ) ;
#5813=VECTOR ( 'NONE', #19084, 1000.000000000000000 ) ;
#5814=CARTESIAN_POINT ( 'NONE',  ( 4.153738564337000838, -77.85351332859899287, -8.713191203520999295 ) ) ;
#5843=CARTESIAN_POINT ( 'NONE',  ( -7.483407197968000801, -77.00000000000000000, 5.437013583706000297 ) ) ;
#5875=VERTEX_POINT ( 'NONE', #46209 ) ;
#5892=DIRECTION ( 'NONE',  ( 0.000000000000000000, 0.7071067811866525998, -0.7071067811864425456 ) ) ;
#5911=ORIENTED_EDGE ( 'NONE', *, *, #32682, .F. ) ;
#5922=CARTESIAN_POINT ( 'NONE',  ( -9.340210362350283901, -76.99999999999998579, 0.02720789100463689644 ) ) ;
#5932=CARTESIAN_POINT ( 'NONE',  ( -0.6017968039497372246, -77.78000000000000114, 9.523103445003338052 ) ) ;
#5937=CARTESIAN_POINT ( 'NONE',  ( -8.997332162609597006, -79.37373539064718386, 3.050007033374654508 ) ) ;
#5960=CARTESIAN_POINT ( 'NONE',  ( 8.538006731470160204, -79.08654938339437024, 4.209831911330708110 ) ) ;
#6016=CARTESIAN_POINT ( 'NONE',  ( -5.773189589619000195, -78.24451001420199248, 8.192511063987998554 ) ) ;
#6032=CARTESIAN_POINT ( 'NONE',  ( -1.184016694733479591, -77.43484693750340853, 9.372457216979636740 ) ) ;
#6035=CARTESIAN_POINT ( 'NONE',  ( 9.342221983604002133, -78.29936001420199432, -2.562053005734000077 ) ) ;
#6054=CARTESIAN_POINT ( 'NONE',  ( 4.145750262472000180, -79.10401332859899526, -8.580453259755000062 ) ) ;
#6059=CARTESIAN_POINT ( 'NONE',  ( -8.997179024602999675, -79.11904514476064776, 3.687079342326999853 ) ) ;
#6063=CARTESIAN_POINT ( 'NONE',  ( -8.630067035710000667, -79.72545584965399712, -4.100810385846999750 ) ) ;
#6069=CARTESIAN_POINT ( 'NONE',  ( 1.243547092045927949, -77.26458333333334849, 9.500000000000003553 ) ) ;
#6070=DIRECTION ( 'NONE',  ( 1.000000000000000000, 0.000000000000000000, 0.000000000000000000 ) ) ;
#6097=EDGE_CURVE ( 'NONE', #9880, #16336, #56791, .T. ) ;
#6098=FACE_BOUND ( 'NONE', #10057, .T. ) ;
#6104=DIRECTION ( 'NONE',  ( 0.000000000000000000, 1.000000000000000000, 0.000000000000000000 ) ) ;
#6121=CARTESIAN_POINT ( 'NONE',  ( -3.339615680726000235, -78.47284805011499031, 9.131854552393999569 ) ) ;
#6137=CARTESIAN_POINT ( 'NONE',  ( -6.722422115750747551, -77.00000000000001421, 6.387398339048315776 ) ) ;
#6164=CARTESIAN_POINT ( 'NONE',  ( 4.897371265365999982, -76.84044415034598785, 7.847181321287999722 ) ) ;
#6182=EDGE_CURVE ( 'NONE', #6658, #11325, #42218, .T. ) ;
#6204=EDGE_LOOP ( 'NONE', ( #41155, #40324, #6266, #38099 ) ) ;
#6223=CARTESIAN_POINT ( 'NONE',  ( -0.8742025125545000996, -78.76128998579800111, 9.984153739810000872 ) ) ;
#6228=CARTESIAN_POINT ( 'NONE',  ( -9.034604909256527705, -79.37471052910895253, 2.936440201109655312 ) ) ;
#6239=DIRECTION ( 'NONE',  ( 0.000000000000000000, 1.000000000000000000, -4.899618830983999950E-14 ) ) ;
#6248=CARTESIAN_POINT ( 'NONE',  ( 7.156381309732353202, -79.10742710526332644, 6.276394420187332734 ) ) ;
#6260=CARTESIAN_POINT ( 'NONE',  ( 6.482950081930999531, -79.37695584965399576, -6.598019266050999754 ) ) ;
#6266=ORIENTED_EDGE ( 'NONE', *, *, #1740, .F. ) ;
#6300=CARTESIAN_POINT ( 'NONE',  ( 6.002077433942410778, -78.07088160286059519, 7.255254208431503038 ) ) ;
#6331=CARTESIAN_POINT ( 'NONE',  ( -7.575359187103000380, -78.51711001420200375, 6.037810896484000267 ) ) ;
#6338=FACE_OUTER_BOUND ( 'NONE', #6898, .T. ) ;
#6349=CARTESIAN_POINT ( 'NONE',  ( 8.557689913033998508, -79.23271332859899019, 4.648766890461000223 ) ) ;
#6354=CARTESIAN_POINT ( 'NONE',  ( 1.899930039692999895, -78.50934514476064408, 9.535935523283001203 ) ) ;
#6357=CARTESIAN_POINT ( 'NONE',  ( 8.395992668097999712, -79.47975584965399776, 4.560928606276999808 ) ) ;
#6362=CARTESIAN_POINT ( 'NONE',  ( -2.486604901413195901, -77.29583333333334849, 9.252740428348989354 ) ) ;
#6373=ORIENTED_EDGE ( 'NONE', *, *, #35099, .T. ) ;
#6378=CARTESIAN_POINT ( 'NONE',  ( 7.552177422520572669, -79.20153084570749513, 5.764790892576884929 ) ) ;
#6388=DIRECTION ( 'NONE',  ( 1.000000000000000000, 0.000000000000000000, 0.000000000000000000 ) ) ;
#6446=CARTESIAN_POINT ( 'NONE',  ( 8.540261029602000065, -76.91613998579799727, 4.257270096473000365 ) ) ;
#6449=EDGE_LOOP ( 'NONE', ( #1746, #16754, #44944 ) ) ;
#6458=B_SPLINE_CURVE_WITH_KNOTS ( 'NONE', 3,
 ( #18405, #13960, #1283, #45865, #36688, #50000, #9546, #54424, #27529, #54703, #55281, #54991, #13666, #14540, #31662, #23407, #32533, #36978, #4825, #4533, #5685, #36396, #40834, #138, #27819, #54125, #27237, #18694, #41122, #26945, #45571, #5118, #428, #23114, #41417 ),
 .UNSPECIFIED., .F., .F.,
 ( 4, 1, 1, 1, 1, 1, 1, 1, 1, 1, 1, 1, 1, 1, 1, 1, 1, 1, 1, 1, 1, 1, 1, 1, 1, 1, 1, 1, 1, 1, 1, 1, 4 ),
 ( 0.000000000000000000, 0.01250096958943576128, 0.04500090495504436433, 0.07750084032066266448, 0.1100007756862671354, 0.1425007110518439757, 0.1750006464174760634, 0.2075005817831081512, 0.2400005171487402389, 0.2725004525143723266, 0.3050003878800044421, 0.3375003232454983904, 0.3700002586111305614, 0.4025001939767626213, 0.4350001293423947368, 0.4675000647080267968, 0.5000000000736588568, 0.5324999354391528605, 0.5649998708047848650, 0.5974998061704170915, 0.6299997415360490960, 0.6624996769016813225, 0.6949996122673132160, 0.7274995476329454425, 0.7599994829984393352, 0.7924994183640715617, 0.8249993537297034552, 0.8574992890953355706, 0.8899992244609679082, 0.9224991598265999126, 0.9549990951922320281, 0.9874990305577258098, 1.000000000000000000 ),
 .UNSPECIFIED. ) ;
#6459=CARTESIAN_POINT ( 'NONE',  ( -5.601841361836865651, -77.97297913613843434, 7.949357391288894625 ) ) ;
#6517=CARTESIAN_POINT ( 'NONE',  ( 8.163677614451000153, -77.67253998579799656, 4.925422544966999716 ) ) ;
#6546=DIRECTION ( 'NONE',  ( -1.044282756598000039E-09, -1.000000000000000000, 6.141137129051000072E-09 ) ) ;
#6557=CARTESIAN_POINT ( 'NONE',  ( 9.722066209057999231, -78.94145584965399109, 0.1588365413100999990 ) ) ;
#6602=CARTESIAN_POINT ( 'NONE',  ( 9.633138876124000660, -78.59291001420200473, 2.765897569310999948 ) ) ;
#6607=EDGE_LOOP ( 'NONE', ( #26105, #44296 ) ) ;
#6616=CARTESIAN_POINT ( 'NONE',  ( -1.937158916668030528, -79.75000000000000000, -9.096604487445336673 ) ) ;
#6622=CARTESIAN_POINT ( 'NONE',  ( 9.525749612248999298, -78.21536332859899687, 2.735063621234999687 ) ) ;
#6635=EDGE_CURVE ( 'NONE', #42830, #44850, #55599, .T. ) ;
#6644=CARTESIAN_POINT ( 'NONE',  ( 9.723265251863999481, -79.19761332859899028, 0.5504220888713000637 ) ) ;
#6658=VERTEX_POINT ( 'NONE', #21559 ) ;
#6673=CARTESIAN_POINT ( 'NONE',  ( 6.169502046027795394, -79.21861551698380310, 7.223965119394421208 ) ) ;
#6676=ORIENTED_EDGE ( 'NONE', *, *, #23431, .F. ) ;
#6694=FACE_OUTER_BOUND ( 'NONE', #20596, .T. ) ;
#6700=CARTESIAN_POINT ( 'NONE',  ( 11.65000000000000036, -76.00000000000000000, 0.000000000000000000 ) ) ;
#6706=CONICAL_SURFACE ( 'NONE', #27422, 1.099999997157999232, 0.7853981633972997312 ) ;
#6712=LINE ( 'NONE', #19420, #33954 ) ;
#6715=B_SPLINE_SURFACE_WITH_KNOTS ( 'NONE', 3, 3, ( 
 ( #34505, #38948, #3519, #12375, #39235, #48405, #29783, #7942, #17679, #25944, #35074, #43386, #12659, #35666, #12091, #47839, #21519, #7370, #30653 ),
 ( #25371, #2945, #56963, #39526, #17091, #52534, #30074, #53111, #25655, #48687, #43684, #3239, #21231, #23280, #49268, #36269, #27982, #14407, #53698 ),
 ( #49574, #4395, #4696, #41577, #54293, #31526, #22395, #23564, #13830, #10003, #2, #40406, #13235, #18856, #53995, #32406, #1158, #46030, #40998 ),
 ( #31229, #9121, #49870, #19146, #54583, #36561, #45736, #14123, #4980, #27693, #8821, #45438, #31828, #869, #50450, #32119, #50160, #5553, #9703 ) ),
 .UNSPECIFIED., .F., .F., .F.,
 ( 4, 4 ),
 ( 4, 1, 1, 1, 1, 1, 1, 1, 1, 1, 1, 1, 1, 1, 1, 1, 4 ),
 ( -0.1377334280162000046, 1.137733428016000081 ),
 ( 0.6650746268656999582, 0.6864179104477999838, 0.7077611940298000892, 0.7291044776119000037, 0.7504477611940000292, 0.7717910447760999437, 0.7931343283582000803, 0.8144776119402999948, 0.8358208955224000203, 0.8571641791044999348, 0.8785074626865999603, 0.8998507462686999858, 0.9211940298506999802, 0.9425373134328000058, 0.9638805970148999203, 0.9852238805970000568, 1.006567164178999940 ),
 .UNSPECIFIED. ) ;
#6748=CARTESIAN_POINT ( 'NONE',  ( 5.102724688570000389, -77.83873581701298860, 7.811319209985999379 ) ) ;
#6754=CARTESIAN_POINT ( 'NONE',  ( -8.920205756585657397, -78.01652913613843054, 3.873438468320558936 ) ) ;
#6807=ORIENTED_EDGE ( 'NONE', *, *, #15995, .F. ) ;
#6854=VECTOR ( 'NONE', #55885, 1000.000000000000000 ) ;
#6871=DIRECTION ( 'NONE',  ( 0.000000000000000000, 1.000000000000000000, 0.000000000000000000 ) ) ;
#6893=B_SPLINE_SURFACE_WITH_KNOTS ( 'NONE', 3, 3, ( 
 ( #48898, #53315, #45058, #12859, #54204, #8438, #40620, #36472, #22011, #40019, #9621, #31739, #58034, #14037, #4611, #217, #53610, #18193, #49783 ),
 ( #9330, #17594, #22307, #13149, #31143, #27320, #32032, #22901, #503, #49184, #50076, #27607, #8735, #26728, #44755, #58333, #17896, #35885, #19641 ),
 ( #23770, #46237, #19353, #9913, #41488, #33498, #46823, #51535, #29071, #28776, #41785, #1650, #50658, #6349, #6644, #32317, #37929, #6054, #19064 ),
 ( #24365, #24653, #10496, #27894, #42377, #1946, #1075, #37640, #42663, #11091, #37346, #45941, #5473, #19940, #18768, #55656, #14616, #14906, #55954 ) ),
 .UNSPECIFIED., .F., .F., .F.,
 ( 4, 4 ),
 ( 4, 1, 1, 1, 1, 1, 1, 1, 1, 1, 1, 1, 1, 1, 1, 1, 4 ),
 ( -0.1377334280162000046, 1.137733428016000081 ),
 ( 0.5889552238806000650, 0.6151492537313000275, 0.6413432835821000211, 0.6675373134327999836, 0.6937313432835999771, 0.7199253731343000506, 0.7461194029851000442, 0.7723134328358000067, 0.7985074626866000003, 0.8247014925372999627, 0.8508955223880999563, 0.8770895522388000298, 0.9032835820896000234, 0.9294776119402999859, 0.9556716417910000594, 0.9818656716417999419, 1.008059701493000171 ),
 .UNSPECIFIED. ) ;
#6895=CARTESIAN_POINT ( 'NONE',  ( -3.403932870613000095, -78.65978667140099390, 9.307723658127001087 ) ) ;
#6898=EDGE_LOOP ( 'NONE', ( #23795, #18909, #40759, #48072 ) ) ;
#6904=CARTESIAN_POINT ( 'NONE',  ( -9.500228589985420413, -79.40182418455218283, -0.2334504967788087748 ) ) ;
#6913=CARTESIAN_POINT ( 'NONE',  ( -5.875581754031000692, -78.86861332859899676, 7.981103691720999649 ) ) ;
#6941=CARTESIAN_POINT ( 'NONE',  ( -9.646692012709998210, -78.63999514476064689, 1.218660606027000215 ) ) ;
#6961=CARTESIAN_POINT ( 'NONE',  ( 9.052015793914058861, -79.17411443971855078, 2.882270040945727363 ) ) ;
#6963=FACE_OUTER_BOUND ( 'NONE', #39975, .T. ) ;
#6976=CARTESIAN_POINT ( 'NONE',  ( -1.983076715186758543, -79.52083333388351605, -9.322644982774999534 ) ) ;
#6982=CARTESIAN_POINT ( 'NONE',  ( 9.499999999999998224, -77.06041666666666856, 1.243547092045980129 ) ) ;
#7013=EDGE_LOOP ( 'NONE', ( #29303, #57828, #58365, #1834, #35011 ) ) ;
#7014=DIRECTION ( 'NONE',  ( 0.7071067811865474617, 0.7071067811865474617, -1.027168298793069202E-09 ) ) ;
#7038=CARTESIAN_POINT ( 'NONE',  ( 5.896171905175000560, -77.86999999999999034, 7.127247495676000355 ) ) ;
#7039=CARTESIAN_POINT ( 'NONE',  ( 6.214091009702999102, -77.69161915034599986, -7.179311535719000048 ) ) ;
#7052=CARTESIAN_POINT ( 'NONE',  ( -4.784380313523539208, -77.98333333333332007, -8.300970689365453126 ) ) ;
#7085=CARTESIAN_POINT ( 'NONE',  ( 9.468750000004000356, -79.53124999999600675, -6.681056941828999630E-10 ) ) ;
#7104=DIRECTION ( 'NONE',  ( -1.000000000000000000, 0.000000000000000000, 0.000000000000000000 ) ) ;
#7137=CARTESIAN_POINT ( 'NONE',  ( -5.600962501326000265, -78.11400584965400640, 7.948110234177999445 ) ) ;
#7183=CARTESIAN_POINT ( 'NONE',  ( -9.042797184480999562, -78.79043667140099672, -4.055650103703999143 ) ) ;
#7200=CARTESIAN_POINT ( 'NONE',  ( -9.721629130303000466, -78.49688667140098630, 1.228127365514999791 ) ) ;
#7223=CARTESIAN_POINT ( 'NONE',  ( 8.500869906239369556, -79.11249999999999716, -4.334382246026802221 ) ) ;
#7232=CARTESIAN_POINT ( 'NONE',  ( -6.090475762158000350, -79.43984415034599067, 7.362120511650999788 ) ) ;
#7251=CARTESIAN_POINT ( 'NONE',  ( 2.890496000096741014, -79.25013075116083883, 9.049465696841215490 ) ) ;
#7327=CARTESIAN_POINT ( 'NONE',  ( 8.386131694562763528, -78.75687913613843705, -4.924049977871809425 ) ) ;
#7370=CARTESIAN_POINT ( 'NONE',  ( 4.163570051248999704, -79.48139334753599883, -8.653020802693998093 ) ) ;
#7385=EDGE_CURVE ( 'NONE', #42268, #22499, #3289, .T. ) ;
#7397=ORIENTED_EDGE ( 'NONE', *, *, #42096, .T. ) ;
#7416=( NAMED_UNIT ( * ) SI_UNIT ( $, .STERADIAN. ) SOLID_ANGLE_UNIT ( ) );
#7427=CARTESIAN_POINT ( 'NONE',  ( -7.603664017118000551, -78.63660584965400346, 6.060370778711000384 ) ) ;
#7464=ORIENTED_EDGE ( 'NONE', *, *, #8298, .T. ) ;
#7465=ORIENTED_EDGE ( 'NONE', *, *, #18739, .F. ) ;
#7474=CARTESIAN_POINT ( 'NONE',  ( -9.786657985941999982, -79.26948667140098337, -1.562668305794999934 ) ) ;
#7492=CARTESIAN_POINT ( 'NONE',  ( -8.940852521590000990, -78.54043667140099672, -4.009928423322000057 ) ) ;
#7498=CARTESIAN_POINT ( 'NONE',  ( 5.838193839761705917, -78.97708333333333997, -7.596835002782701629 ) ) ;
#7505=DIRECTION ( 'NONE',  ( 0.000000000000000000, 1.000000000000000000, 4.744707668127999788E-14 ) ) ;
#7517=ADVANCED_FACE ( 'NONE', ( #7996 ), #5013, .F. ) ;
#7531=CARTESIAN_POINT ( 'NONE',  ( -2.486604901413195456, -78.69583333333335418, 9.252740428348991131 ) ) ;
#7542=CARTESIAN_POINT ( 'NONE',  ( 2.946058150294987410, -79.24962501036633000, 9.031517904169495736 ) ) ;
#7546=ORIENTED_EDGE ( 'NONE', *, *, #55086, .T. ) ;
#7548=CARTESIAN_POINT ( 'NONE',  ( 4.044903269867999640, -79.46000000000000796, -8.595856998426999240 ) ) ;
#7571=CARTESIAN_POINT ( 'NONE',  ( 0.000000000000000000, -74.70999999999999375, 0.000000000000000000 ) ) ;
#7623=CARTESIAN_POINT ( 'NONE',  ( 7.596835002782719393, -78.09791666666666288, -5.838193839761677495 ) ) ;
#7627=CARTESIAN_POINT ( 'NONE',  ( -5.838193839761721016, -78.82708333333333428, 7.596835002782687418 ) ) ;
#7633=CARTESIAN_POINT ( 'NONE',  ( 0.000000000000000000, -75.20000000000000284, -7.200000000000000178 ) ) ;
#7660=ORIENTED_EDGE ( 'NONE', *, *, #52934, .T. ) ;
#7697=B_SPLINE_CURVE_WITH_KNOTS ( 'NONE', 3,
 ( #27028, #4617, #40627, #46827, #52113, #11096, #6059, #33789, #51539, #24659, #28781, #42964, #2521, #50952, #24370, #20523, #55661, #6941, #38521, #56536, #6354, #2809, #56250, #1952, #42382, #42086, #11386, #37646, #10800, #2237, #42669, #10502, #29076, #33503, #16097 ),
 .UNSPECIFIED., .F., .F.,
 ( 4, 1, 1, 1, 1, 1, 1, 1, 1, 1, 1, 1, 1, 1, 1, 1, 1, 1, 1, 1, 1, 1, 1, 1, 1, 1, 1, 1, 1, 1, 1, 1, 4 ),
 ( 0.000000000000000000, 0.01250353271130624083, 0.04500329721509613301, 0.07750306171888603213, 0.1100028262226759312, 0.1425025907264658165, 0.1750023552302557295, 0.2075021197340456147, 0.2400018842378355277, 0.2725016487416254685, 0.3050014132454152982, 0.3375011777492052389, 0.3700009422529951242, 0.4025007067567850649, 0.4350004712605748947, 0.4675002357643648354, 0.5000000002681546096, 0.5324997647719444949, 0.5649995292757343801, 0.5974992937795243764, 0.6299990582833142616, 0.6624988227871041468, 0.6949985872908940321, 0.7274983517946840283, 0.7599981162984738026, 0.7924978808022636878, 0.8249976453060535730, 0.8574974098098435693, 0.8899971743136334545, 0.9224969388174233398, 0.9549967033212132250, 0.9874964678250032213, 1.000000000000000000 ),
 .UNSPECIFIED. ) ;
#7711=CARTESIAN_POINT ( 'NONE',  ( 2.858407197969000002, -77.00000000000000000, 8.797272775729998884 ) ) ;
#7715=CARTESIAN_POINT ( 'NONE',  ( 7.048436826466999428, -77.93776861655099708, 6.223291978577000449 ) ) ;
#7721=DIRECTION ( 'NONE',  ( 0.000000000000000000, 1.000000000000000000, 0.000000000000000000 ) ) ;
#7731=FACE_OUTER_BOUND ( 'NONE', #57988, .T. ) ;
#7741=CARTESIAN_POINT ( 'NONE',  ( 5.894914467206975317, -77.90333333333336441, 7.125729969419699827 ) ) ;
#7755=EDGE_LOOP ( 'NONE', ( #1326, #57184, #32739, #54055 ) ) ;
#7760=CARTESIAN_POINT ( 'NONE',  ( -0.6596342590195000133, -78.13718667140099683, 9.888746480308999054 ) ) ;
#7801=CARTESIAN_POINT ( 'NONE',  ( 9.500000000000001776, -79.14249999999998408, -0.8953539062730788700 ) ) ;
#7811=CARTESIAN_POINT ( 'NONE',  ( 4.067416459488999436, -79.23084805011500009, -8.418325902196000854 ) ) ;
#7830=CARTESIAN_POINT ( 'NONE',  ( -5.496009875325862382, -79.32396257907269899, 7.748915864499907435 ) ) ;
#7847=CARTESIAN_POINT ( 'NONE',  ( -5.694495468273999883, -77.08086167140099576, -7.629186780306000060 ) ) ;
#7865=CARTESIAN_POINT ( 'NONE',  ( 0.000000000000000000, -75.00000000000000000, -8.399999999999769429 ) ) ;
#7871=DIRECTION ( 'NONE',  ( 1.000000000000000000, 0.000000000000000000, 0.000000000000000000 ) ) ;
#7909=CARTESIAN_POINT ( 'NONE',  ( 9.230360848053999590, -77.48048667140099610, -3.179709793684999841 ) ) ;
#7942=CARTESIAN_POINT ( 'NONE',  ( -6.862551019151999832, -79.75786001420199511, 6.914489430668000480 ) ) ;
#7953=EDGE_CURVE ( 'NONE', #49594, #49808, #28561, .T. ) ;
#7964=CARTESIAN_POINT ( 'NONE',  ( 8.979348251287998295, -77.96650584965399844, 3.086914251890999772 ) ) ;
#7968=PRODUCT_DEFINITION_CONTEXT ( 'detailed design', #28888, 'design' ) ;
#7996=FACE_OUTER_BOUND ( 'NONE', #8393, .T. ) ;
#8002=CARTESIAN_POINT ( 'NONE',  ( -9.601739433208001273, -79.08254805011499400, -1.533141744029000053 ) ) ;
#8043=CARTESIAN_POINT ( 'NONE',  ( 2.202483111904999902, -79.27258998579800675, -9.433251486511000650 ) ) ;
#8048=ORIENTED_EDGE ( 'NONE', *, *, #17294, .T. ) ;
#8049=VERTEX_POINT ( 'NONE', #31196 ) ;
#8053=CARTESIAN_POINT ( 'NONE',  ( -8.300970689365447797, -77.44166666666666288, -4.784380313523547201 ) ) ;
#8056=CARTESIAN_POINT ( 'NONE',  ( -4.947170628245625146, -79.48109446742806483, -8.109985010457963384 ) ) ;
#8106=CARTESIAN_POINT ( 'NONE',  ( -7.596835002782738933, -78.74791666666668277, 5.838193839761661508 ) ) ;
#8107=DIRECTION ( 'NONE',  ( -1.000000000000000000, 0.000000000000000000, 0.000000000000000000 ) ) ;
#8118=CARTESIAN_POINT ( 'NONE',  ( -3.689560173563782630, -79.30639694791827310, 8.754108420648137212 ) ) ;
#8126=DIRECTION ( 'NONE',  ( 0.7071067811865975328, -0.7071067811864976127, -1.396793747092993108E-09 ) ) ;
#8136=VECTOR ( 'NONE', #26641, 1000.000000000000114 ) ;
#8163=DIRECTION ( 'NONE',  ( 0.000000000000000000, 1.000000000000000000, 0.000000000000000000 ) ) ;
#8172=ORIENTED_EDGE ( 'NONE', *, *, #5380, .T. ) ;
#8179=AXIS2_PLACEMENT_3D ( 'NONE', #30707, #13585, #49625 ) ;
#8192=CARTESIAN_POINT ( 'NONE',  ( -9.083128614440136417, -79.67447916666266394, 2.440148008508001620 ) ) ;
#8199=CARTESIAN_POINT ( 'NONE',  ( -0.1226781409794000105, -77.88088667140100085, -9.761919256278002166 ) ) ;
#8254=CARTESIAN_POINT ( 'NONE',  ( 6.214091009702999102, -77.87193084965399237, -7.179311535719000048 ) ) ;
#8285=CARTESIAN_POINT ( 'NONE',  ( 4.518822441307924542, -77.00000000000000000, 8.100777538286340729 ) ) ;
#8288=CARTESIAN_POINT ( 'NONE',  ( 2.013632425233999879, -78.33175584965400162, -9.512575055159999238 ) ) ;
#8298=EDGE_CURVE ( 'NONE', #31756, #15737, #9795, .T. ) ;
#8323=CARTESIAN_POINT ( 'NONE',  ( 3.670568130644999982, -77.97173998579799559, 8.453023018411998990 ) ) ;
#8330=CARTESIAN_POINT ( 'NONE',  ( 9.342221983604002133, -78.35803998579800123, -2.562053005734000077 ) ) ;
#8342=CARTESIAN_POINT ( 'NONE',  ( -8.991148217401329745, -79.42591775919153463, -3.068505234713029051 ) ) ;
#8357=CARTESIAN_POINT ( 'NONE',  ( -9.252740428348994683, -78.32083333333335418, -2.486604901413163926 ) ) ;
#8379=CARTESIAN_POINT ( 'NONE',  ( 9.199999999999999289, -79.79999999999999716, 0.000000000000000000 ) ) ;
#8393=EDGE_LOOP ( 'NONE', ( #55972, #52073, #32992, #33298 ) ) ;
#8403=CARTESIAN_POINT ( 'NONE',  ( 1.470118532801963473, -79.26259840585061056, 9.385540567805065848 ) ) ;
#8404=ORIENTED_EDGE ( 'NONE', *, *, #21135, .T. ) ;
#8436=CARTESIAN_POINT ( 'NONE',  ( 0.9983493978779336420, -79.03333333333330302, -9.480860074790918191 ) ) ;
#8438=CARTESIAN_POINT ( 'NONE',  ( -6.030860253222999567, -79.64106001420199732, -7.365124455302999529 ) ) ;
#8439=CARTESIAN_POINT ( 'NONE',  ( 0.000000000000000000, -75.20000000000000284, 0.000000000000000000 ) ) ;
#8475=CARTESIAN_POINT ( 'NONE',  ( -2.455355391147715061, -79.62239583332932114, 9.133204103880812497 ) ) ;
#8485=CARTESIAN_POINT ( 'NONE',  ( 9.762601837900000135, -77.00728667140100470, 0.04909978866182999196 ) ) ;
#8510=DIRECTION ( 'NONE',  ( -1.000000000000000000, 0.000000000000000000, 0.000000000000000000 ) ) ;
#8564=CARTESIAN_POINT ( 'NONE',  ( 3.967828918824999995, -77.10191332859899660, -8.773065546720999919 ) ) ;
#8577=CARTESIAN_POINT ( 'NONE',  ( 7.990874060778157428, -76.99999999999998579, 4.858782514301908328 ) ) ;
#8580=CARTESIAN_POINT ( 'NONE',  ( -0.6471704932797999188, -77.89014415034598926, 9.701898969124000516 ) ) ;
#8584=VERTEX_POINT ( 'NONE', #22451 ) ;
#8585=DIRECTION ( 'NONE',  ( -1.000000000000000000, 0.000000000000000000, 0.000000000000000000 ) ) ;
#8621=CARTESIAN_POINT ( 'NONE',  ( 7.981661899572999985, -77.98631332859899601, 4.815606314103999530 ) ) ;
#8631=CARTESIAN_POINT ( 'NONE',  ( 9.252740428349001789, -77.62916666666666288, -2.486604901413144830 ) ) ;
#8635=CARTESIAN_POINT ( 'NONE',  ( -9.023370604008427165, -79.42502604630486474, -2.970777336590622930 ) ) ;
#8655=CARTESIAN_POINT ( 'NONE',  ( -11.44999999995999929, -74.99999999996167332, -1.667681223830999978E-09 ) ) ;
#8700=CARTESIAN_POINT ( 'NONE',  ( -1.506252837058942529, -79.28748717942596613, 9.379723702719340750 ) ) ;
#8729=AXIS2_PLACEMENT_3D ( 'NONE', #29528, #20688, #21256 ) ;
#8735=CARTESIAN_POINT ( 'NONE',  ( 5.689140600256999747, -79.33158667140099851, 7.768672748409000128 ) ) ;
#8774=CARTESIAN_POINT ( 'NONE',  ( 9.462239583424770117, -79.53776041666264973, 1.239456475944461955 ) ) ;
#8784=CARTESIAN_POINT ( 'NONE',  ( 5.016617212972000139, -78.02337999526599788, 7.984403404948999139 ) ) ;
#8821=CARTESIAN_POINT ( 'NONE',  ( 2.751744599267999636, -79.48073998579799593, 9.005047869058000032 ) ) ;
#8827=VERTEX_POINT ( 'NONE', #56818 ) ;
#8842=CARTESIAN_POINT ( 'NONE',  ( -9.391369684923001060, -77.17838084965399048, 1.399863080762999923 ) ) ;
#8854=CARTESIAN_POINT ( 'NONE',  ( 9.252740428348991131, -77.57083333333333997, 2.486604901413179913 ) ) ;
#8862=CARTESIAN_POINT ( 'NONE',  ( -1.661399596109000010, -77.55431332859899385, -9.484202486144001298 ) ) ;
#8872=CARTESIAN_POINT ( 'NONE',  ( 6.540748709914804948, -77.00000000000001421, 6.638316095770077752 ) ) ;
#8874=CARTESIAN_POINT ( 'NONE',  ( 4.495978696100999983, -77.84659415034599306, 8.621246072682998474 ) ) ;
#8896=FACE_OUTER_BOUND ( 'NONE', #19477, .T. ) ;
#8897=EDGE_CURVE ( 'NONE', #15380, #10154, #54744, .T. ) ;
#8913=CARTESIAN_POINT ( 'NONE',  ( -7.118194945375000415, -77.57133998579800505, 6.355464284701999311 ) ) ;
#8914=ORIENTED_EDGE ( 'NONE', *, *, #54145, .T. ) ;
#8932=CARTESIAN_POINT ( 'NONE',  ( -7.632609106719096204, -79.45061835715877407, -5.673732696205357584 ) ) ;
#8940=VERTEX_POINT ( 'NONE', #9550 ) ;
#8969=DIRECTION ( 'NONE',  ( 0.000000000000000000, -1.000000000000000000, 0.000000000000000000 ) ) ;
#8970=EDGE_CURVE ( 'NONE', #45023, #16336, #1230, .T. ) ;
#8985=DIRECTION ( 'NONE',  ( 0.000000000000000000, -1.000000000000000000, 0.000000000000000000 ) ) ;
#9000=CARTESIAN_POINT ( 'NONE',  ( -5.740620664195313694, -79.32657994115034228, 7.569668994968869136 ) ) ;
#9005=DIRECTION ( 'NONE',  ( 0.000000000000000000, 1.000000000000000000, 0.000000000000000000 ) ) ;
#9010=B_SPLINE_CURVE_WITH_KNOTS ( 'NONE', 3,
 ( #35283, #22009, #58032, #8436, #26431, #30282, #22305, #26725, #44753, #57452, #4305, #52739, #4004, #57735, #40320, #12291, #34994, #57160 ),
 .UNSPECIFIED., .F., .F.,
 ( 4, 2, 2, 2, 2, 2, 2, 2, 4 ),
 ( 0.000000000000000000, 0.1249999999999999167, 0.2499999999999998890, 0.3749999999999998335, 0.4999999999999998890, 0.6249999999999998890, 0.7499999999999998890, 0.8750000000000000000, 1.000000000000000000 ),
 .UNSPECIFIED. ) ;
#9020=B_SPLINE_CURVE_WITH_KNOTS ( 'NONE', 3,
 ( #52222, #51942, #2065, #42786, #2916, #7627, #25628, #52505, #28898, #38340, #15622, #21200, #51661, #11209, #33326, #30043, #11779, #34474 ),
 .UNSPECIFIED., .F., .F.,
 ( 4, 2, 2, 2, 2, 2, 2, 2, 4 ),
 ( 0.000000000000000000, 0.1249999999999998335, 0.2499999999999997224, 0.3749999999999997224, 0.4999999999999997780, 0.6249999999999997780, 0.7499999999999998890, 0.8749999999999998890, 1.000000000000000000 ),
 .UNSPECIFIED. ) ;
#9083=CARTESIAN_POINT ( 'NONE',  ( 9.545926504039998761, -77.99008667140098794, -2.045769860731999845 ) ) ;
#9096=AXIS2_PLACEMENT_3D ( 'NONE', #42485, #56065, #29742 ) ;
#9121=CARTESIAN_POINT ( 'NONE',  ( -2.944350850530000230, -79.72860665246399492, -8.802063698512000656 ) ) ;
#9122=DIRECTION ( 'NONE',  ( 1.000000000000000000, 0.000000000000000000, 0.000000000000000000 ) ) ;
#9140=CARTESIAN_POINT ( 'NONE',  ( 5.807838419657000095, -77.24732305011499989, -7.511754867730999763 ) ) ;
#9158=CARTESIAN_POINT ( 'NONE',  ( 8.270412359550473269, -77.00833333333331154, -4.779119312162220190 ) ) ;
#9162=CARTESIAN_POINT ( 'NONE',  ( -1.680129511012999899, -77.49053998579799440, -9.591123365327000272 ) ) ;
#9169=DIRECTION ( 'NONE',  ( 0.000000000000000000, 0.000000000000000000, -1.000000000000000000 ) ) ;
#9171=CARTESIAN_POINT ( 'NONE',  ( 8.492816448344902014, -77.00000000000001421, -4.278825844373149501 ) ) ;
#9173=CARTESIAN_POINT ( 'NONE',  ( -5.764562846862999912, -78.93534415034599760, 7.830301022820999712 ) ) ;
#9186=ORIENTED_EDGE ( 'NONE', *, *, #58236, .F. ) ;
#9194=VECTOR ( 'NONE', #29876, 1000.000000000000000 ) ;
#9204=CARTESIAN_POINT ( 'NONE',  ( -4.784380313523539208, -78.48333333333332007, -8.300970689365453126 ) ) ;
#9207=ORIENTED_EDGE ( 'NONE', *, *, #25617, .F. ) ;
#9212=CARTESIAN_POINT ( 'NONE',  ( 6.644622036202999737, -78.31448998579800502, -7.049129409659999901 ) ) ;
#9226=CARTESIAN_POINT ( 'NONE',  ( -8.469455166620191378, -79.43739211172909620, -4.303251210716531716 ) ) ;
#9292=CARTESIAN_POINT ( 'NONE',  ( -7.748038516948378529, -79.35049307451645006, 5.497056738179014523 ) ) ;
#9319=EDGE_LOOP ( 'NONE', ( #17864, #38888, #11473, #34810 ) ) ;
#9330=CARTESIAN_POINT ( 'NONE',  ( 8.213537570112000807, -79.71768667140099751, -4.408490834274999770 ) ) ;
#9359=CARTESIAN_POINT ( 'NONE',  ( 9.445921377069225855, -79.15851891711977828, 1.025770609074986961 ) ) ;
#9369=EDGE_CURVE ( 'NONE', #15380, #25723, #1968, .T. ) ;
#9380=CARTESIAN_POINT ( 'NONE',  ( -1.281965430112000037, -77.30751332859900060, -9.567121928242999118 ) ) ;
#9434=CARTESIAN_POINT ( 'NONE',  ( 8.256620083228000340, -77.27884805011498770, -4.688888258373000717 ) ) ;
#9455=CARTESIAN_POINT ( 'NONE',  ( 7.170910619513000128, -77.68846498579799231, 6.587124128982000393 ) ) ;
#9464=CARTESIAN_POINT ( 'NONE',  ( 9.089938076053588389, -77.00000000000001421, 2.444550776227857991 ) ) ;
#9466=CARTESIAN_POINT ( 'NONE',  ( 8.384816012895999648, -78.77769805011500637, -4.923277454554000343 ) ) ;
#9491=CIRCLE ( 'NONE', #37759, 11.65000000000000036 ) ;
#9546=CARTESIAN_POINT ( 'NONE',  ( 6.214091009702999102, -77.83177403538302030, -7.179311535718999160 ) ) ;
#9550=CARTESIAN_POINT ( 'NONE',  ( 5.299999999999999822, -75.00000000000000000, 0.000000000000000000 ) ) ;
#9552=CARTESIAN_POINT ( 'NONE',  ( 2.865789910122292561, -79.75000000000000000, -8.824825250167616986 ) ) ;
#9578=ORIENTED_EDGE ( 'NONE', *, *, #32734, .T. ) ;
#9581=DIRECTION ( 'NONE',  ( 0.000000000000000000, 0.7071067811866525998, -0.7071067811864425456 ) ) ;
#9599=DIRECTION ( 'NONE',  ( 1.000000000000000000, 0.000000000000000000, 0.000000000000000000 ) ) ;
#9603=CARTESIAN_POINT ( 'NONE',  ( 4.581254438705999910, -78.73486001420198477, -8.535416510302999527 ) ) ;
#9621=CARTESIAN_POINT ( 'NONE',  ( -2.355755099258999508, -79.46556001420199777, 9.223161221019999800 ) ) ;
#9649=CARTESIAN_POINT ( 'NONE',  ( 9.368176195122705607, -79.16304405940145728, 1.578867174401747064 ) ) ;
#9664=CARTESIAN_POINT ( 'NONE',  ( 5.165981523686999921, -77.89863501420200009, 7.709125646902999840 ) ) ;
#9666=CARTESIAN_POINT ( 'NONE',  ( 0.000000000000000000, -75.00000000000000000, 0.000000000000000000 ) ) ;
#9667=CARTESIAN_POINT ( 'NONE',  ( 0.000000000000000000, -75.00000000000000000, -5.300000000000069988 ) ) ;
#9686=CARTESIAN_POINT ( 'NONE',  ( 0.000000000000000000, -80.79999999999999716, 0.000000000000000000 ) ) ;
#9703=CARTESIAN_POINT ( 'NONE',  ( 2.979603836623999857, -79.28053998579800066, -8.720586535794000227 ) ) ;
#9724=CARTESIAN_POINT ( 'NONE',  ( 4.574312611392000072, -77.46505194988499454, 8.320643751074999983 ) ) ;
#9731=ORIENTED_EDGE ( 'NONE', *, *, #24108, .T. ) ;
#9732=CARTESIAN_POINT ( 'NONE',  ( 1.243547092045928615, -77.66458333333332575, 9.500000000000003553 ) ) ;
#9743=CARTESIAN_POINT ( 'NONE',  ( 5.316634094433000612, -77.27156332859900090, 8.027686297795002091 ) ) ;
#9779=CARTESIAN_POINT ( 'NONE',  ( -8.563626910508329360, -77.00000000000001421, -3.884937692711959656 ) ) ;
#9790=CARTESIAN_POINT ( 'NONE',  ( 4.739769873023999658, -78.54353998579799168, -8.830749431300999319 ) ) ;
#9795=B_SPLINE_CURVE_WITH_KNOTS ( 'NONE', 3,
 ( #44970, #17811, #8357, #4526, #22818, #48527, #54119, #22225, #35202, #22526, #40536, #40829, #26639, #57658, #131, #31360, #18108, #35797 ),
 .UNSPECIFIED., .F., .F.,
 ( 4, 2, 2, 2, 2, 2, 2, 2, 4 ),
 ( 0.000000000000000000, 0.1250000000000000833, 0.2500000000000001665, 0.3750000000000002220, 0.5000000000000002220, 0.6250000000000002220, 0.7500000000000001110, 0.8750000000000001110, 1.000000000000000000 ),
 .UNSPECIFIED. ) ;
#9797=VECTOR ( 'NONE', #46076, 1000.000000000000114 ) ;
#9813=DIRECTION ( 'NONE',  ( 1.000000000000000000, 0.000000000000000000, 0.000000000000000000 ) ) ;
#9817=CARTESIAN_POINT ( 'NONE',  ( 9.249780780301254168, -79.07089109199264954, 2.485615031187831558 ) ) ;
#9837=CIRCLE ( 'NONE', #52263, 1.199999999999999956 ) ;
#9876=VECTOR ( 'NONE', #41806, 1000.000000000000000 ) ;
#9880=VERTEX_POINT ( 'NONE', #12629 ) ;
#9895=CARTESIAN_POINT ( 'NONE',  ( 6.559997675027998909, -78.38646001420198672, 7.127949055663999722 ) ) ;
#9900=DIRECTION ( 'NONE',  ( 0.000000000000000000, -1.000000000000000000, 0.000000000000000000 ) ) ;
#9913=CARTESIAN_POINT ( 'NONE',  ( 1.896935383555999888, -79.58371332859898928, -9.552341775358000220 ) ) ;
#9923=CARTESIAN_POINT ( 'NONE',  ( 8.857115352654000517, -79.34945194988499395, -3.584237475251999872 ) ) ;
#9937=EDGE_CURVE ( 'NONE', #39245, #45676, #14993, .T. ) ;
#9949=LINE ( 'NONE', #10832, #26173 ) ;
#9960=CARTESIAN_POINT ( 'NONE',  ( 2.142412200439999914, -77.42738501420200237, 9.164433333602998388 ) ) ;
#9961=FACE_OUTER_BOUND ( 'NONE', #37952, .T. ) ;
#9975=CARTESIAN_POINT ( 'NONE',  ( -1.000000000000000000, -75.20000000000000284, -7.200000000000000178 ) ) ;
#10003=CARTESIAN_POINT ( 'NONE',  ( -0.5980611300388000151, -79.57311332859899267, 9.505909450771000024 ) ) ;
#10008=DIRECTION ( 'NONE',  ( 0.000000000000000000, -1.000000000000000000, 0.000000000000000000 ) ) ;
#10012=FACE_OUTER_BOUND ( 'NONE', #6204, .T. ) ;
#10022=CARTESIAN_POINT ( 'NONE',  ( -4.342561293556999935, -77.71725194988499652, -8.443909622126001935 ) ) ;
#10031=CARTESIAN_POINT ( 'NONE',  ( 9.199999999968001774, -80.60000000003199716, -3.388768808660000233E-10 ) ) ;
#10041=ADVANCED_FACE ( 'NONE', ( #32804 ), #30974, .F. ) ;
#10057=EDGE_LOOP ( 'NONE', ( #9186, #29101 ) ) ;
#10087=CARTESIAN_POINT ( 'NONE',  ( 6.682297893293000612, -79.06613998579798874, -6.800905403285999462 ) ) ;
#10154=VERTEX_POINT ( 'NONE', #35409 ) ;
#10156=DIRECTION ( 'NONE',  ( 0.000000000000000000, 0.000000000000000000, 1.000000000000000000 ) ) ;
#10189=CARTESIAN_POINT ( 'NONE',  ( -7.502741683071000089, -78.12516001420199530, -6.127813063941999872 ) ) ;
#10212=CARTESIAN_POINT ( 'NONE',  ( 7.507056363060000237, -79.82915194988498797, -5.572808305725000189 ) ) ;
#10216=CARTESIAN_POINT ( 'NONE',  ( 4.888751005523273463, -79.67187500068790484, -7.978256377688620837 ) ) ;
#10217=CIRCLE ( 'NONE', #58293, 9.199999999999999289 ) ;
#10235=CARTESIAN_POINT ( 'NONE',  ( 0.000000000000000000, -75.10000000284179578, 6.100000002841999169 ) ) ;
#10253=CARTESIAN_POINT ( 'NONE',  ( 0.000000000000000000, -79.66562500002999059, 0.000000000000000000 ) ) ;
#10257=CARTESIAN_POINT ( 'NONE',  ( 2.223069596159087169, -77.04374999999998863, -9.266319061195876117 ) ) ;
#10313=CARTESIAN_POINT ( 'NONE',  ( 9.475051992780000987, -77.87487694988500664, -0.6170397550469999270 ) ) ;
#10320=VERTEX_POINT ( 'NONE', #30911 ) ;
#10335=CIRCLE ( 'NONE', #52726, 1.199999999999999956 ) ;
#10344=VERTEX_POINT ( 'NONE', #56652 ) ;
#10361=CARTESIAN_POINT ( 'NONE',  ( -8.888234858626997692, -77.00000000000000000, -2.992064833292889858 ) ) ;
#10370=CARTESIAN_POINT ( 'NONE',  ( 4.582566119076999733, -77.77986332859900642, 8.787281441338999244 ) ) ;
#10377=CARTESIAN_POINT ( 'NONE',  ( -9.099455430112048049, -79.37646600500266914, 2.730131614506341009 ) ) ;
#10394=CARTESIAN_POINT ( 'NONE',  ( -7.941067684623824618, -79.34731494385309247, -5.274242742192593703 ) ) ;
#10416=ORIENTED_EDGE ( 'NONE', *, *, #58012, .T. ) ;
#10424=CARTESIAN_POINT ( 'NONE',  ( 3.552101903221845713, -79.75000000000000000, -8.571631383469688004 ) ) ;
#10425=LINE ( 'NONE', #14255, #6854 ) ;
#10450=VERTEX_POINT ( 'NONE', #1130 ) ;
#10456=CARTESIAN_POINT ( 'NONE',  ( -9.927618387633998509, -78.33161001420199909, -1.374747298418999897 ) ) ;
#10472=CARTESIAN_POINT ( 'NONE',  ( -4.765392682094479859, -77.63277193750339222, -8.156953009811001465 ) ) ;
#10476=CARTESIAN_POINT ( 'NONE',  ( 2.202483111904999902, -79.21391001420199984, -9.433251486511000650 ) ) ;
#10491=VECTOR ( 'NONE', #41802, 1000.000000000000000 ) ;
#10496=CARTESIAN_POINT ( 'NONE',  ( 5.858810443405999990, -79.55503998579798974, -7.916359134618999427 ) ) ;
#10502=CARTESIAN_POINT ( 'NONE',  ( -0.6471704932797999188, -78.03029514476064321, 9.701898969124000516 ) ) ;
#10503=AXIS2_PLACEMENT_3D ( 'NONE', #11762, #47512, #28590 ) ;
#10507=CARTESIAN_POINT ( 'NONE',  ( -2.364557222828000072, -79.46484805011499475, 9.257622954664000758 ) ) ;
#10511=CARTESIAN_POINT ( 'NONE',  ( 0.7412195882237281319, -79.57812500151310076, -9.421874992337064825 ) ) ;
#10526=CARTESIAN_POINT ( 'NONE',  ( 9.491245595196989626, -79.15441013100512180, 0.5281570930040961898 ) ) ;
#10544=CARTESIAN_POINT ( 'NONE',  ( 6.931088847199000647, -77.87978501420199962, 6.366826336012000098 ) ) ;
#10551=CARTESIAN_POINT ( 'NONE',  ( -3.620936601582000147, -77.59871332859898985, 8.947741361997000098 ) ) ;
#10563=CARTESIAN_POINT ( 'NONE',  ( 9.722066209057999231, -78.82124805011498836, 0.1588365413100999990 ) ) ;
#10585=ORIENTED_EDGE ( 'NONE', *, *, #44937, .T. ) ;
#10600=EDGE_LOOP ( 'NONE', ( #20585, #56275, #40903, #17611 ) ) ;
#10601=CARTESIAN_POINT ( 'NONE',  ( 1.199999999999999956, -75.00000000000000000, 7.200000000000000178 ) ) ;
#10607=CARTESIAN_POINT ( 'NONE',  ( 1.009320482739999969, -77.37636915034599383, 9.441330439200999791 ) ) ;
#10618=CARTESIAN_POINT ( 'NONE',  ( 9.500000000000000000, -78.14999999999999147, 0.000000000000000000 ) ) ;
#10627=EDGE_LOOP ( 'NONE', ( #30384, #50389, #33597, #41007 ) ) ;
#10671=CARTESIAN_POINT ( 'NONE',  ( -9.312500000004000356, -79.68749999999599254, 6.570867420027000168E-10 ) ) ;
#10674=CARTESIAN_POINT ( 'NONE',  ( 7.265173101945999967, -77.68705665246400827, 6.414655419558000560 ) ) ;
#10678=CARTESIAN_POINT ( 'NONE',  ( -8.833271293965303528, -79.36966988906971210, 3.510040627682449177 ) ) ;
#10732=AXIS2_PLACEMENT_3D ( 'NONE', #48758, #3875, #39883 ) ;
#10743=AXIS2_PLACEMENT_3D ( 'NONE', #25782, #43808, #20779 ) ;
#10757=CARTESIAN_POINT ( 'NONE',  ( -7.629208874607999569, -79.37681001420199323, -6.499394396314999156 ) ) ;
#10772=CARTESIAN_POINT ( 'NONE',  ( 9.416651550578160723, -77.29347193750339784, -0.7559916624287352782 ) ) ;
#10776=CARTESIAN_POINT ( 'NONE',  ( 7.022198843594999573, -77.87837668086899612, 6.200125618097000135 ) ) ;
#10800=CARTESIAN_POINT ( 'NONE',  ( -9.631455446501000495, -78.16094514476064603, -1.333735528292999906 ) ) ;
#10814=CARTESIAN_POINT ( 'NONE',  ( 0.000000000000000000, -76.79999999999999716, 0.000000000000000000 ) ) ;
#10826=CARTESIAN_POINT ( 'NONE',  ( 8.730844907503701791, -79.18198688127804985, 3.749782986556219111 ) ) ;
#10832=CARTESIAN_POINT ( 'NONE',  ( -1.199999995321999968, -75.00000000467838390, 7.199999972488000388 ) ) ;
#10836=CARTESIAN_POINT ( 'NONE',  ( 0.000000000000000000, -80.79999999999999716, 0.000000000000000000 ) ) ;
#10844=CARTESIAN_POINT ( 'NONE',  ( -7.901745553563000790, -77.11636001420200159, -5.112651159007999269 ) ) ;
#10880=CARTESIAN_POINT ( 'NONE',  ( 2.858407197969000002, -77.00000000000000000, 8.797272775729998884 ) ) ;
#10884=VERTEX_POINT ( 'NONE', #43233 ) ;
#10897=CARTESIAN_POINT ( 'NONE',  ( -9.522203062526999773, -77.13453998579799986, -0.6231167251167999410 ) ) ;
#10925=EDGE_CURVE ( 'NONE', #35206, #45023, #34349, .T. ) ;
#10964=CARTESIAN_POINT ( 'NONE',  ( -3.442307367123000450, -78.28223998579800025, 9.412654989800000038 ) ) ;
#10990=SURFACE_STYLE_USAGE ( .BOTH. , #33689 ) ;
#11023=CIRCLE ( 'NONE', #32673, 1.199999999999999956 ) ;
#11070=AXIS2_PLACEMENT_3D ( 'NONE', #55942, #15492, #37917 ) ;
#11072=CARTESIAN_POINT ( 'NONE',  ( 1.936520525790000002, -78.30246332859900349, 9.719586767747999900 ) ) ;
#11078=CYLINDRICAL_SURFACE ( 'NONE', #17514, 9.500000000000000000 ) ;
#11091=CARTESIAN_POINT ( 'NONE',  ( -6.277755163971999508, -79.30933998579799038, 7.588502419953999656 ) ) ;
#11096=CARTESIAN_POINT ( 'NONE',  ( -9.601739433208001273, -79.16259514476064396, -1.533141744029000053 ) ) ;
#11100=CARTESIAN_POINT ( 'NONE',  ( 2.769824414688999870, -79.33935584965399812, -8.825563591736999669 ) ) ;
#11104=CARTESIAN_POINT ( 'NONE',  ( -4.784380313523575623, -77.31666666666666288, 8.300970689365433586 ) ) ;
#11120=CARTESIAN_POINT ( 'NONE',  ( 9.040019095898385260, -79.17444713763063646, 2.919477139292010914 ) ) ;
#11135=CYLINDRICAL_SURFACE ( 'NONE', #12749, 9.199999999999999289 ) ;
#11140=CARTESIAN_POINT ( 'NONE',  ( -4.802278608554999551, -77.58981167140099444, -8.220090885098999323 ) ) ;
#11148=FACE_OUTER_BOUND ( 'NONE', #48847, .T. ) ;
#11173=ORIENTED_EDGE ( 'NONE', *, *, #17233, .T. ) ;
#11188=CARTESIAN_POINT ( 'NONE',  ( -6.301614265331000553, -77.06173998579799900, 7.165911196006999440 ) ) ;
#11196=CARTESIAN_POINT ( 'NONE',  ( -9.454379850511999805, -77.50246915034600192, 0.8787206290761000460 ) ) ;
#11199=CARTESIAN_POINT ( 'NONE',  ( 3.938458446976999205, -79.21000000000000796, -8.369650235310999165 ) ) ;
#11209=CARTESIAN_POINT ( 'NONE',  ( 7.596835002782696300, -78.70208333333332007, 5.838193839761711246 ) ) ;
#11234=ORIENTED_EDGE ( 'NONE', *, *, #12558, .T. ) ;
#11254=VERTEX_POINT ( 'NONE', #17816 ) ;
#11297=DIRECTION ( 'NONE',  ( -1.000000000000000000, 0.000000000000000000, 0.000000000000000000 ) ) ;
#11316=AXIS2_PLACEMENT_3D ( 'NONE', #28119, #18703, #50297 ) ;
#11325=VERTEX_POINT ( 'NONE', #52272 ) ;
#11336=CARTESIAN_POINT ( 'NONE',  ( -8.940852521590000990, -78.72666332859900251, -4.009928423322000057 ) ) ;
#11339=EDGE_CURVE ( 'NONE', #23790, #8940, #52718, .T. ) ;
#11356=CARTESIAN_POINT ( 'NONE',  ( 4.686931394918000038, -78.60731332859899112, -8.732305124302000010 ) ) ;
#11367=DIRECTION ( 'NONE',  ( -1.000000000000000000, 0.000000000000000000, 0.000000000000000000 ) ) ;
#11386=CARTESIAN_POINT ( 'NONE',  ( -3.230363664242999810, -78.24804514476065265, -9.171071524558000121 ) ) ;
#11404=CARTESIAN_POINT ( 'NONE',  ( 8.925046886613115404, -79.17747656854896832, 3.256041339590551420 ) ) ;
#11421=CARTESIAN_POINT ( 'NONE',  ( 2.167121982807000080, -77.36361167140100292, 9.270132485773999065 ) ) ;
#11435=CYLINDRICAL_SURFACE ( 'NONE', #26997, 9.500000000000000000 ) ;
#11457=LINE ( 'NONE', #25592, #22065 ) ;
#11463=B_SPLINE_CURVE_WITH_KNOTS ( 'NONE', 3,
 ( #28196, #51548, #24952, #55375, #46835, #5776, #11104, #6362, #24378, #6069, #42677, #2246, #55083, #24077, #20243, #1370, #38236, #15808 ),
 .UNSPECIFIED., .F., .F.,
 ( 4, 2, 2, 2, 2, 2, 2, 2, 4 ),
 ( 0.000000000000000000, 0.1249999999999998335, 0.2499999999999997224, 0.3749999999999997224, 0.4999999999999997780, 0.6249999999999997780, 0.7499999999999998890, 0.8749999999999998890, 1.000000000000000000 ),
 .UNSPECIFIED. ) ;
#11473=ORIENTED_EDGE ( 'NONE', *, *, #32253, .F. ) ;
#11476=CARTESIAN_POINT ( 'NONE',  ( -8.818477034137000459, -77.09813998579799943, 3.646243024668999855 ) ) ;
#11483=CARTESIAN_POINT ( 'NONE',  ( -7.264520526674999701, -77.56551915034600597, -6.114261184555999762 ) ) ;
#11493=CARTESIAN_POINT ( 'NONE',  ( -8.706831144604571193, -79.33395239776687902, -3.878314185012179838 ) ) ;
#11501=MECHANICAL_DESIGN_GEOMETRIC_PRESENTATION_REPRESENTATION('',(#20917),#51915);
#11515=CARTESIAN_POINT ( 'NONE',  ( -2.935661446561999899, -77.00000000000000000, -9.035036904803998681 ) ) ;
#11519=AXIS2_PLACEMENT_3D ( 'NONE', #20480, #11629, #56780 ) ;
#11528=CARTESIAN_POINT ( 'NONE',  ( 9.473958333266658371, -79.52604166666334606, -0.9915651818467657863 ) ) ;
#11579=CARTESIAN_POINT ( 'NONE',  ( 6.669449228234999971, -78.37530584965399783, -7.075468016816000016 ) ) ;
#11589=EDGE_CURVE ( 'NONE', #10884, #4309, #107, .T. ) ;
#11597=DIRECTION ( 'NONE',  ( -3.655298286142000429E-11, 1.000000000000000000, 1.590757531940000291E-09 ) ) ;
#11627=CARTESIAN_POINT ( 'NONE',  ( 8.377812017747999107, -79.05173667140100235, 5.294595800518999695 ) ) ;
#11629=DIRECTION ( 'NONE',  ( 0.000000000000000000, -1.000000000000000000, 0.000000000000000000 ) ) ;
#11645=CARTESIAN_POINT ( 'NONE',  ( -7.675809325333999844, -77.99761332859900165, -6.269164879585000349 ) ) ;
#11653=CARTESIAN_POINT ( 'NONE',  ( 0.000000000000000000, -75.20000000000000284, -7.200000000000000178 ) ) ;
#11693=CARTESIAN_POINT ( 'NONE',  ( 3.575328375144039228, -79.24388340919793450, 8.805561371781996272 ) ) ;
#11714=CARTESIAN_POINT ( 'NONE',  ( -9.252740428349008894, -77.27916666666671119, 2.486604901413127955 ) ) ;
#11762=CARTESIAN_POINT ( 'NONE',  ( 0.000000000000000000, -74.70999999999999375, 0.000000000000000000 ) ) ;
#11766=CARTESIAN_POINT ( 'NONE',  ( -0.8482561879233938562, -78.93107913613843607, 9.687824124670456172 ) ) ;
#11778=DIRECTION ( 'NONE',  ( 0.000000000000000000, 1.000000000000000000, 0.000000000000000000 ) ) ;
#11779=CARTESIAN_POINT ( 'NONE',  ( 9.500000000000001776, -78.66041666666667709, 1.243547092045981239 ) ) ;
#11815=CARTESIAN_POINT ( 'NONE',  ( -9.051338284747782126, -77.00000000000000000, 2.171493758094802828 ) ) ;
#11817=ADVANCED_FACE ( 'NONE', ( #36731 ), #31930, .F. ) ;
#11820=ORIENTED_EDGE ( 'NONE', *, *, #11589, .F. ) ;
#11821=ORIENTED_EDGE ( 'NONE', *, *, #32253, .T. ) ;
#11837=DIRECTION ( 'NONE',  ( 0.000000000000000000, 1.000000000000000000, 0.000000000000000000 ) ) ;
#11847=DIRECTION ( 'NONE',  ( 0.000000000000000000, 1.000000000000000000, 0.000000000000000000 ) ) ;
#11866=CARTESIAN_POINT ( 'NONE',  ( 6.669449228234999971, -78.31520194988499384, -7.075468016816000016 ) ) ;
#11906=CARTESIAN_POINT ( 'NONE',  ( -3.098141882180000195, -79.35658667140100420, -9.414028956051998520 ) ) ;
#11927=CARTESIAN_POINT ( 'NONE',  ( -0.5414817640998000892, -78.56376332859900913, -9.895821147420001296 ) ) ;
#11933=CARTESIAN_POINT ( 'NONE',  ( 9.500000000000005329, -79.03958333333333997, -1.243547092045939939 ) ) ;
#11944=VECTOR ( 'NONE', #22743, 1000.000000000000114 ) ;
#11963=CARTESIAN_POINT ( 'NONE',  ( -9.500000000000000000, -77.29999999999999716, 0.000000000000000000 ) ) ;
#11976=ORIENTED_EDGE ( 'NONE', *, *, #29217, .T. ) ;
#11978=CARTESIAN_POINT ( 'NONE',  ( 3.065954117407362123, -79.24853233248634865, 8.991551369834709817 ) ) ;
#11994=CARTESIAN_POINT ( 'NONE',  ( -0.9882926363948538739, -79.54166666776707473, -9.458333340432636405 ) ) ;
#12027=EDGE_CURVE ( 'NONE', #10154, #9880, #36035, .T. ) ;
#12051=CARTESIAN_POINT ( 'NONE',  ( -0.6472720423598817829, -77.92942913613843814, 9.703421317447949335 ) ) ;
#12059=CARTESIAN_POINT ( 'NONE',  ( 4.248461405734000884, -77.98106001420198652, -8.911888886500999973 ) ) ;
#12091=CARTESIAN_POINT ( 'NONE',  ( 9.612200201122000465, -79.55766001420199984, -1.584397442130999867 ) ) ;
#12109=FACE_OUTER_BOUND ( 'NONE', #52758, .T. ) ;
#12119=DIRECTION ( 'NONE',  ( -1.000000000000000000, 0.000000000000000000, 0.000000000000000000 ) ) ;
#12146=CARTESIAN_POINT ( 'NONE',  ( 4.495978696100999983, -77.96680194988499579, 8.621246072682998474 ) ) ;
#12180=FILL_AREA_STYLE ('',( #3040 ) ) ;
#12184=ORIENTED_EDGE ( 'NONE', *, *, #20894, .T. ) ;
#12193=CARTESIAN_POINT ( 'NONE',  ( 2.253288347564000205, -79.40013667140100040, -9.650850687256999905 ) ) ;
#12229=CARTESIAN_POINT ( 'NONE',  ( 4.044903269867999640, -79.05999999999998806, -8.595856998426999240 ) ) ;
#12258=CARTESIAN_POINT ( 'NONE',  ( 0.1752985264899695750, -79.27328162838476544, 9.505737417831570113 ) ) ;
#12291=CARTESIAN_POINT ( 'NONE',  ( -9.399464885765262068, -78.91333333333335531, -1.591687513073350990 ) ) ;
#12313=ORIENTED_EDGE ( 'NONE', *, *, #45487, .F. ) ;
#12342=CARTESIAN_POINT ( 'NONE',  ( -3.662222950988999859, -77.66248667140099826, 9.049764572265999618 ) ) ;
#12375=CARTESIAN_POINT ( 'NONE',  ( -7.764665820177000022, -79.87226001420199850, -5.883443353344000037 ) ) ;
#12379=ADVANCED_FACE ( 'NONE', ( #5003 ), #5574, .T. ) ;
#12416=CARTESIAN_POINT ( 'NONE',  ( 9.342458652602138258, -77.03333333333333144, -1.989514594393971603 ) ) ;
#12417=CARTESIAN_POINT ( 'NONE',  ( 0.9999999970759999579, -75.20000000292399989, -7.199999982805000087 ) ) ;
#12431=CONICAL_SURFACE ( 'NONE', #2093, 5.199999999809000073, 0.7853981633972997312 ) ;
#12434=CARTESIAN_POINT ( 'NONE',  ( 6.482950081930999531, -79.25674805011499302, -6.598019266050999754 ) ) ;
#12459=CARTESIAN_POINT ( 'NONE',  ( 0.9999999970759999579, -75.20000000292399989, 7.200000017194999380 ) ) ;
#12470=CARTESIAN_POINT ( 'NONE',  ( -9.816946295765999864, -78.26783667140099965, -1.359421753724999959 ) ) ;
#12479=CARTESIAN_POINT ( 'NONE',  ( -1.243547092045951263, -77.51458333333332007, -9.500000000000003553 ) ) ;
#12483=CARTESIAN_POINT ( 'NONE',  ( -6.722882011319116558, -79.46222606496974095, -6.711992429377692915 ) ) ;
#12525=DIRECTION ( 'NONE',  ( 0.000000000000000000, -1.000000000000000000, 0.000000000000000000 ) ) ;
#12532=CARTESIAN_POINT ( 'NONE',  ( 9.500000000000000000, -78.54999999999999716, 0.000000000000000000 ) ) ;
#12535=ORIENTED_EDGE ( 'NONE', *, *, #12904, .F. ) ;
#12538=ORIENTED_EDGE ( 'NONE', *, *, #47199, .F. ) ;
#12544=CARTESIAN_POINT ( 'NONE',  ( -1.627038676344989110, -79.28854989600672809, 9.360266054361467525 ) ) ;
#12545=VERTEX_POINT ( 'NONE', #27285 ) ;
#12558=EDGE_CURVE ( 'NONE', #52926, #39245, #16867, .T. ) ;
#12560=AXIS2_PLACEMENT_3D ( 'NONE', #41259, #18829, #47873 ) ;
#12626=CARTESIAN_POINT ( 'NONE',  ( 7.000738396026999766, -77.01039334753599519, -6.633884475650999590 ) ) ;
#12629=CARTESIAN_POINT ( 'NONE',  ( 9.500000000000000000, -77.64999999999999147, 0.000000000000000000 ) ) ;
#12659=CARTESIAN_POINT ( 'NONE',  ( 8.277425028854000999, -79.61486001420199443, 5.137022432363000490 ) ) ;
#12680=CARTESIAN_POINT ( 'NONE',  ( 7.092659876394000307, -77.93792694988499647, 6.312768414564000174 ) ) ;
#12715=CARTESIAN_POINT ( 'NONE',  ( -5.505695391233000002, -78.70715194988498808, -8.014431902511001127 ) ) ;
#12720=CARTESIAN_POINT ( 'NONE',  ( -9.500000000000000000, -78.29999999999999716, 0.000000000000000000 ) ) ;
#12737=CARTESIAN_POINT ( 'NONE',  ( -9.000000000000000000, -80.79999999999999716, 0.000000000000000000 ) ) ;
#12749=AXIS2_PLACEMENT_3D ( 'NONE', #47450, #1992, #43001 ) ;
#12755=CARTESIAN_POINT ( 'NONE',  ( 7.890654042133999901, -77.92253998579799656, 4.760698198672999482 ) ) ;
#12758=ORIENTED_EDGE ( 'NONE', *, *, #22057, .F. ) ;
#12766=CARTESIAN_POINT ( 'NONE',  ( -6.899571484722149428, -79.46005502588960212, -6.530559442748636201 ) ) ;
#12793=CARTESIAN_POINT ( 'NONE',  ( 9.500000000000000000, -77.54999999999999716, 0.000000000000000000 ) ) ;
#12814=CARTESIAN_POINT ( 'NONE',  ( -9.252740428349008894, -78.77916666666668277, 2.486604901413127955 ) ) ;
#12815=CARTESIAN_POINT ( 'NONE',  ( 0.000000000000000000, -79.79999999999999716, 0.000000000000000000 ) ) ;
#12827=CARTESIAN_POINT ( 'NONE',  ( -3.727509208301453381, -79.30673376728708490, 8.737982862341825196 ) ) ;
#12843=STYLED_ITEM ( 'NONE', ( #15407 ), #17895 ) ;
#12859=CARTESIAN_POINT ( 'NONE',  ( 1.854164892466000136, -79.71126001420199714, -9.336963670056000808 ) ) ;
#12904=EDGE_CURVE ( 'NONE', #14353, #37723, #31979, .T. ) ;
#12907=CARTESIAN_POINT ( 'NONE',  ( 6.877190604583000244, -77.44408667140099567, -6.929239867807000408 ) ) ;
#12913=CARTESIAN_POINT ( 'NONE',  ( -8.650571159592999493, -79.61510095943374665, 4.057379972786000266 ) ) ;
#12953=ADVANCED_FACE ( 'NONE', ( #50120 ), #17234, .F. ) ;
#12977=CARTESIAN_POINT ( 'NONE',  ( 8.727615157005653046, -77.01666666666665151, -3.881808298730416773 ) ) ;
#12981=CARTESIAN_POINT ( 'NONE',  ( -9.207228400713001193, -77.40571498579799936, -3.168505599523000260 ) ) ;
#12988=DIRECTION ( 'NONE',  ( 0.000000000000000000, 0.000000000000000000, -1.000000000000000000 ) ) ;
#12997=CARTESIAN_POINT ( 'NONE',  ( 6.669449228234999971, -78.19499415034600531, -7.075468016816000016 ) ) ;
#13030=CARTESIAN_POINT ( 'NONE',  ( 7.596835002782719393, -78.59791666666667709, -5.838193839761677495 ) ) ;
#13031=CARTESIAN_POINT ( 'NONE',  ( -9.378008371271000954, -77.64413998579800591, -1.764535237813999791 ) ) ;
#13038=CARTESIAN_POINT ( 'NONE',  ( 4.479242302639000251, -77.96608998579800698, 8.589153267943999026 ) ) ;
#13046=CARTESIAN_POINT ( 'NONE',  ( 7.596835002782719393, -77.59791666666664867, -5.838193839761677495 ) ) ;
#13050=CARTESIAN_POINT ( 'NONE',  ( -9.384480618050281109, -79.41205795043663329, -1.475605007748509223 ) ) ;
#13055=CARTESIAN_POINT ( 'NONE',  ( -4.209390496675390558, -79.21181571460809323, 8.537567007200664193 ) ) ;
#13097=AXIS2_PLACEMENT_3D ( 'NONE', #27575, #54747, #759 ) ;
#13104=ORIENTED_EDGE ( 'NONE', *, *, #1527, .T. ) ;
#13114=CARTESIAN_POINT ( 'NONE',  ( -1.479726591698317328, -79.28725347445197258, 9.383940043454046531 ) ) ;
#13129=CARTESIAN_POINT ( 'NONE',  ( 5.896171905175000560, -77.86999999999999034, 7.127247495676000355 ) ) ;
#13149=CARTESIAN_POINT ( 'NONE',  ( 1.875550138011000012, -79.64748667140099769, -9.444652722706999626 ) ) ;
#13198=CARTESIAN_POINT ( 'NONE',  ( 3.712903092914000336, -78.03551332859899503, 8.550517029640001709 ) ) ;
#13206=CARTESIAN_POINT ( 'NONE',  ( 4.789894294226004767, -79.31810081118388212, -7.967628558423081486 ) ) ;
#13225=FACE_OUTER_BOUND ( 'NONE', #21824, .T. ) ;
#13235=CARTESIAN_POINT ( 'NONE',  ( 8.092873224492999285, -79.48731332859900078, 5.022488412950999681 ) ) ;
#13257=DIRECTION ( 'NONE',  ( 1.000000000000000000, 0.000000000000000000, 0.000000000000000000 ) ) ;
#13278=CARTESIAN_POINT ( 'NONE',  ( 4.339214180343000216, -77.71673998579798592, 8.489796212882000148 ) ) ;
#13289=CARTESIAN_POINT ( 'NONE',  ( 6.134715390259300349, -76.99999999999998579, 6.994583833444441012 ) ) ;
#13291=CARTESIAN_POINT ( 'NONE',  ( -8.871933854994999535, -78.54339415034600336, -3.979018739998999354 ) ) ;
#13298=CARTESIAN_POINT ( 'NONE',  ( -9.500000000000003553, -78.29250000000001819, 0.8953539062730667686 ) ) ;
#13336=ORIENTED_EDGE ( 'NONE', *, *, #37501, .F. ) ;
#13345=CARTESIAN_POINT ( 'NONE',  ( -8.487831271174274050, -79.43705601822802009, -4.266955699134562074 ) ) ;
#13370=EDGE_CURVE ( 'NONE', #11254, #43096, #4567, .T. ) ;
#13398=ORIENTED_EDGE ( 'NONE', *, *, #8970, .T. ) ;
#13403=ORIENTED_EDGE ( 'NONE', *, *, #31084, .T. ) ;
#13411=CARTESIAN_POINT ( 'NONE',  ( -3.597607681491937992, -79.30558875575349020, 8.792251918324103244 ) ) ;
#13426=CARTESIAN_POINT ( 'NONE',  ( 9.489539964980000519, -77.25051167140100006, -0.7618433214053000890 ) ) ;
#13469=ORIENTED_EDGE ( 'NONE', *, *, #27416, .F. ) ;
#13490=LINE ( 'NONE', #41826, #56013 ) ;
#13498=CARTESIAN_POINT ( 'NONE',  ( 4.201099985035000373, -77.91728667140098707, -8.812540045011001411 ) ) ;
#13555=ORIENTED_EDGE ( 'NONE', *, *, #22813, .T. ) ;
#13556=CARTESIAN_POINT ( 'NONE',  ( 1.009320482739999969, -77.43647305011499782, 9.441330439200999791 ) ) ;
#13575=CARTESIAN_POINT ( 'NONE',  ( -9.625876801520000470, -77.44121332859899098, 0.2298721198045000080 ) ) ;
#13585=DIRECTION ( 'NONE',  ( 0.000000000000000000, 1.000000000000000000, 0.000000000000000000 ) ) ;
#13591=CARTESIAN_POINT ( 'NONE',  ( -7.541360678298865139, -78.24750000000000227, 5.846326858574210306 ) ) ;
#13593=CIRCLE ( 'NONE', #23962, 9.000000000000000000 ) ;
#13620=CARTESIAN_POINT ( 'NONE',  ( -4.321547818559999143, -77.71693998579799256, -8.507928659197000698 ) ) ;
#13640=CARTESIAN_POINT ( 'NONE',  ( 9.500000000000001776, -77.63958333333334849, -1.243547092045940827 ) ) ;
#13643=CARTESIAN_POINT ( 'NONE',  ( -9.382059563581934825, -79.41218430702922149, -1.490898798910053724 ) ) ;
#13648=CARTESIAN_POINT ( 'NONE',  ( -8.301610278666615272, -79.25879058881317007, 4.784404709358717867 ) ) ;
#13650=ORIENTED_EDGE ( 'NONE', *, *, #15995, .T. ) ;
#13666=CARTESIAN_POINT ( 'NONE',  ( -9.454379850511999805, -77.64262403538302237, 0.8787206290761000460 ) ) ;
#13670=CARTESIAN_POINT ( 'NONE',  ( 9.252740428349003565, -77.52916666666668277, -2.486604901413146607 ) ) ;
#13697=EDGE_CURVE ( 'NONE', #10344, #24467, #31079, .T. ) ;
#13707=CARTESIAN_POINT ( 'NONE',  ( -9.405479261938486601, -79.38837580768372959, 1.346545511743854506 ) ) ;
#13722=FACE_OUTER_BOUND ( 'NONE', #17398, .T. ) ;
#13742=ORIENTED_EDGE ( 'NONE', *, *, #44937, .F. ) ;
#13750=DIRECTION ( 'NONE',  ( 0.000000000000000000, -1.000000000000000000, 0.000000000000000000 ) ) ;
#13771=VERTEX_POINT ( 'NONE', #806 ) ;
#13789=CARTESIAN_POINT ( 'NONE',  ( 3.074963689382999910, -77.34391332859900103, -9.149746207635999440 ) ) ;
#13828=VERTEX_POINT ( 'NONE', #4852 ) ;
#13830=CARTESIAN_POINT ( 'NONE',  ( -3.903182590741000269, -79.60171332859900417, 8.688219438824999585 ) ) ;
#13834=FACE_OUTER_BOUND ( 'NONE', #46094, .T. ) ;
#13851=CARTESIAN_POINT ( 'NONE',  ( 7.092659876394000307, -77.87782305011499773, 6.312768414564000174 ) ) ;
#13852=B_SPLINE_CURVE_WITH_KNOTS ( 'NONE', 3,
 ( #17098, #35082, #53118, #52737, #48604, #34420, #51879, #33842, #38859, #24997, #25858, #21143, #39443, #20286, #15856, #16436, #24715, #48040 ),
 .UNSPECIFIED., .F., .F.,
 ( 4, 2, 2, 2, 2, 2, 2, 2, 4 ),
 ( 0.000000000000000000, 0.1249999999999998335, 0.2499999999999997224, 0.3749999999999997224, 0.4999999999999997780, 0.6249999999999997780, 0.7499999999999998890, 0.8749999999999998890, 1.000000000000000000 ),
 .UNSPECIFIED. ) ;
#13872=CARTESIAN_POINT ( 'NONE',  ( -9.398705699948999737, -76.96053832859900012, -2.091559270920000380 ) ) ;
#13883=CARTESIAN_POINT ( 'NONE',  ( 6.669449228234999971, -78.25509805011499509, -7.075468016816000016 ) ) ;
#13926=CARTESIAN_POINT ( 'NONE',  ( -8.651034356561854821, -79.51480282387936427, 4.057597226198490503 ) ) ;
#13960=CARTESIAN_POINT ( 'NONE',  ( 6.257930884930855697, -77.96595801179425678, 6.827456521059489525 ) ) ;
#13964=CARTESIAN_POINT ( 'NONE',  ( 6.055527902613000002, -77.71999999999999886, 7.319875806370000682 ) ) ;
#13992=ORIENTED_EDGE ( 'NONE', *, *, #33434, .F. ) ;
#13999=DIRECTION ( 'NONE',  ( 0.000000000000000000, 1.000000000000000000, -5.913433368273000022E-14 ) ) ;
#14004=CARTESIAN_POINT ( 'NONE',  ( 0.000000000000000000, -80.59999999999999432, 0.000000000000000000 ) ) ;
#14017=CARTESIAN_POINT ( 'NONE',  ( -3.028287605162000240, -79.17036001420198943, -9.201769410957998829 ) ) ;
#14033=B_SPLINE_CURVE_WITH_KNOTS ( 'NONE', 3,
 ( #2787, #42652, #20221, #37626 ),
 .UNSPECIFIED., .F., .F.,
 ( 4, 4 ),
 ( 0.000000000000000000, 1.000000000000000000 ),
 .UNSPECIFIED. ) ;
#14036=AXIS2_PLACEMENT_3D ( 'NONE', #14004, #9005, #45907 ) ;
#14037=CARTESIAN_POINT ( 'NONE',  ( 8.364738374805998689, -79.36026001420199805, 4.543950435144999744 ) ) ;
#14053=CARTESIAN_POINT ( 'NONE',  ( 0.000000000000000000, -75.00000000000000000, 0.000000000000000000 ) ) ;
#14055=ORIENTED_EDGE ( 'NONE', *, *, #33434, .T. ) ;
#14123=CARTESIAN_POINT ( 'NONE',  ( -6.633041932324000634, -79.56653998579798781, 6.683243331267000542 ) ) ;
#14135=CARTESIAN_POINT ( 'NONE',  ( 0.000000000000000000, -75.20000000000000284, 7.200000000000000178 ) ) ;
#14139=CARTESIAN_POINT ( 'NONE',  ( -9.391369684923001060, -77.05817305011500196, 1.399863080762999923 ) ) ;
#14153=AXIS2_PLACEMENT_3D ( 'NONE', #17670, #22081, #35656 ) ;
#14158=CARTESIAN_POINT ( 'NONE',  ( 4.012560540388999009, -77.03813998579801137, -8.871969369447000986 ) ) ;
#14167=CARTESIAN_POINT ( 'NONE',  ( 8.130366562757448179, -77.00000000000001421, -4.953553662479941444 ) ) ;
#14175=LINE ( 'NONE', #643, #48359 ) ;
#14202=CARTESIAN_POINT ( 'NONE',  ( 8.472259919707001430, -78.67418998579800871, 5.354284829591000161 ) ) ;
#14216=CIRCLE ( 'NONE', #23661, 5.100000000000000533 ) ;
#14247=CARTESIAN_POINT ( 'NONE',  ( 9.500000000000000000, -78.04999999999999716, 0.000000000000000000 ) ) ;
#14255=CARTESIAN_POINT ( 'NONE',  ( -0.9999999970759999579, -75.20000000292399989, 7.199999982805000087 ) ) ;
#14287=B_SPLINE_CURVE_WITH_KNOTS ( 'NONE', 3,
 ( #22456, #35428, #49337, #3866, #57886, #58180, #36030, #17442, #4455, #54056, #49038, #35733, #13591, #40166, #4160, #35141, #13298, #12720 ),
 .UNSPECIFIED., .F., .F.,
 ( 4, 2, 2, 2, 2, 2, 2, 2, 4 ),
 ( 0.000000000000000000, 0.1250000000000000555, 0.2500000000000001110, 0.3750000000000001665, 0.5000000000000002220, 0.6250000000000001110, 0.7500000000000001110, 0.8750000000000000000, 1.000000000000000000 ),
 .UNSPECIFIED. ) ;
#14300=CARTESIAN_POINT ( 'NONE',  ( -1.630052463839491317, -77.66104693750340004, -9.305255440227826469 ) ) ;
#14305=CARTESIAN_POINT ( 'NONE',  ( -0.8547114690830001082, -78.88883667140099476, 9.761549055228000427 ) ) ;
#14336=DIRECTION ( 'NONE',  ( 0.000000000000000000, -1.000000000000000000, 0.000000000000000000 ) ) ;
#14353=VERTEX_POINT ( 'NONE', #34227 ) ;
#14368=CARTESIAN_POINT ( 'NONE',  ( 5.225564025660000667, -77.83486167140100065, 7.798039823611999211 ) ) ;
#14376=CARTESIAN_POINT ( 'NONE',  ( 9.411694425802703989, -77.13749999999998863, -1.492218284488986191 ) ) ;
#14407=CARTESIAN_POINT ( 'NONE',  ( 4.117154990835999229, -79.41762000473400462, -8.556557796581000019 ) ) ;
#14412=CARTESIAN_POINT ( 'NONE',  ( 0.000000000000000000, -74.70999999999999375, 0.000000000000000000 ) ) ;
#14425=ORIENTED_EDGE ( 'NONE', *, *, #24530, .T. ) ;
#14430=CARTESIAN_POINT ( 'NONE',  ( -9.204193785523999694, -77.08969805011498977, -2.332437886131999871 ) ) ;
#14447=CARTESIAN_POINT ( 'NONE',  ( 0.000000000000000000, -74.70999999999999375, 0.000000000000000000 ) ) ;
#14455=ORIENTED_EDGE ( 'NONE', *, *, #51935, .T. ) ;
#14459=CARTESIAN_POINT ( 'NONE',  ( 0.000000000000000000, -74.70999999999999375, 0.000000000000000000 ) ) ;
#14495=CARTESIAN_POINT ( 'NONE',  ( -0.6670706960860000034, -77.75963998579798897, 10.00022801703000042 ) ) ;
#14508=EDGE_LOOP ( 'NONE', ( #13336, #29308, #34033, #25292 ) ) ;
#14540=CARTESIAN_POINT ( 'NONE',  ( -8.383077572658999443, -77.61109903538302035, 4.458862939031999595 ) ) ;
#14549=EDGE_CURVE ( 'NONE', #89, #41814, #36571, .T. ) ;
#14564=DIRECTION ( 'NONE',  ( 1.000000000000000000, 0.000000000000000000, 0.000000000000000000 ) ) ;
#14577=CARTESIAN_POINT ( 'NONE',  ( -3.442307367123000450, -78.72356001420199334, 9.412654989800000038 ) ) ;
#14580=LINE ( 'NONE', #19318, #40443 ) ;
#14583=ORIENTED_EDGE ( 'NONE', *, *, #8897, .T. ) ;
#14598=CARTESIAN_POINT ( 'NONE',  ( -9.565996717342001077, -79.08326001420199702, -1.527434585433000036 ) ) ;
#14612=VECTOR ( 'NONE', #25995, 1000.000000000000000 ) ;
#14616=CARTESIAN_POINT ( 'NONE',  ( 6.678307047331999868, -79.06363998579800523, -7.238412584370999880 ) ) ;
#14626=CARTESIAN_POINT ( 'NONE',  ( -8.650571159592999493, -79.65525584965399730, 4.057379972786000266 ) ) ;
#14646=ORIENTED_EDGE ( 'NONE', *, *, #42170, .T. ) ;
#14658=CARTESIAN_POINT ( 'NONE',  ( 1.702514374278000009, -77.71013501420199532, -9.256252642129998875 ) ) ;
#14718=CARTESIAN_POINT ( 'NONE',  ( -2.712012240502000182, -77.52810194988499859, 9.099584490865000319 ) ) ;
#14772=CARTESIAN_POINT ( 'NONE',  ( -6.226806355049928854, -76.99999999999998579, -7.114065959849781073 ) ) ;
#14783=CARTESIAN_POINT ( 'NONE',  ( -9.896988620242000323, -78.89193998579798972, -1.580285165976000217 ) ) ;
#14790=CARTESIAN_POINT ( 'NONE',  ( -9.469866204336648607, -79.39351776117217696, 0.7547688023506700095 ) ) ;
#14796=CYLINDRICAL_SURFACE ( 'NONE', #16190, 9.500000000000000000 ) ;
#14820=CARTESIAN_POINT ( 'NONE',  ( -5.764562846862999912, -79.11565584965399012, 7.830301022820999712 ) ) ;
#14837=CARTESIAN_POINT ( 'NONE',  ( 1.924380748938630393E-07, -79.75000000000001421, -9.249538042332323684 ) ) ;
#14843=ADVANCED_FACE ( 'NONE', ( #4082, #13225 ), #4685, .T. ) ;
#14856=CARTESIAN_POINT ( 'NONE',  ( 6.055527902613000002, -78.11999999999999034, 7.319875806370000682 ) ) ;
#14866=CARTESIAN_POINT ( 'NONE',  ( 2.075550720420999973, -78.46226001420198770, -9.805082477504999616 ) ) ;
#14892=DIRECTION ( 'NONE',  ( -1.000000000000000000, 0.000000000000000000, 0.000000000000000000 ) ) ;
#14906=CARTESIAN_POINT ( 'NONE',  ( 4.192487693857999353, -79.04023998579799581, -8.677185653192001524 ) ) ;
#14916=CARTESIAN_POINT ( 'NONE',  ( -2.317989000404999889, -79.67544805011499420, -9.269382932261999386 ) ) ;
#14922=ORIENTED_EDGE ( 'NONE', *, *, #8897, .F. ) ;
#14933=ORIENTED_EDGE ( 'NONE', *, *, #39148, .F. ) ;
#14954=CARTESIAN_POINT ( 'NONE',  ( 8.713118354389999709, -77.85151001420200600, 3.557876713735000251 ) ) ;
#14957=CARTESIAN_POINT ( 'NONE',  ( 9.500000000000000000, -77.04999999999999716, 0.000000000000000000 ) ) ;
#14960=CARTESIAN_POINT ( 'NONE',  ( 7.359424254351999650, -77.99911332859899460, 6.245857008621999107 ) ) ;
#14963=CARTESIAN_POINT ( 'NONE',  ( 6.187590335240950701, -77.08125000000001137, -7.247098261820500653 ) ) ;
#14972=CARTESIAN_POINT ( 'NONE',  ( 6.584508673715999905, -78.32564415034599392, 7.154582167228999978 ) ) ;
#14993=CIRCLE ( 'NONE', #48922, 9.199999999999999289 ) ;
#15017=CARTESIAN_POINT ( 'NONE',  ( 8.503129636637000388, -77.72314415034598767, -4.225430575863000193 ) ) ;
#15068=DIRECTION ( 'NONE',  ( 0.000000000000000000, -1.000000000000000000, 0.000000000000000000 ) ) ;
#15082=ORIENTED_EDGE ( 'NONE', *, *, #27863, .F. ) ;
#15132=EDGE_CURVE ( 'NONE', #34146, #49594, #45517, .T. ) ;
#15146=VERTEX_POINT ( 'NONE', #85 ) ;
#15153=CARTESIAN_POINT ( 'NONE',  ( 5.896171905175000560, -77.96999999999999886, 7.127247495676000355 ) ) ;
#15179=CARTESIAN_POINT ( 'NONE',  ( -2.858407197967999913, -79.75000000000000000, -8.797272775729998884 ) ) ;
#15182=CARTESIAN_POINT ( 'NONE',  ( -8.775882267141646764, -77.51967193750340357, 3.496961574127103400 ) ) ;
#15187=CARTESIAN_POINT ( 'NONE',  ( 4.479242302639000251, -77.90741001420200007, 8.589153267943999026 ) ) ;
#15214=CARTESIAN_POINT ( 'NONE',  ( 5.645287065787000458, -79.51485584965399767, 7.708789581145000014 ) ) ;
#15219=CARTESIAN_POINT ( 'NONE',  ( 5.492755654603074689, -79.68750000055037219, -7.555491173184210929 ) ) ;
#15233=CARTESIAN_POINT ( 'NONE',  ( 1.574959781464393860, -79.26172491759977845, 9.368679406100806517 ) ) ;
#15293=EDGE_LOOP ( 'NONE', ( #49754, #45436, #48422, #14455 ) ) ;
#15311=ORIENTED_EDGE ( 'NONE', *, *, #17826, .T. ) ;
#15316=CARTESIAN_POINT ( 'NONE',  ( -1.269916711065999904, -77.12416915034599185, -9.409822520238998678 ) ) ;
#15321=CARTESIAN_POINT ( 'NONE',  ( 4.599093535406832522, -78.71332913613842663, -8.568652848198281546 ) ) ;
#15330=B_SPLINE_CURVE_WITH_KNOTS ( 'NONE', 3,
 ( #42897, #25739, #7741, #21027 ),
 .UNSPECIFIED., .F., .F.,
 ( 4, 4 ),
 ( 0.000000000000000000, 1.000000000000000000 ),
 .UNSPECIFIED. ) ;
#15339=ORIENTED_EDGE ( 'NONE', *, *, #1740, .T. ) ;
#15380=VERTEX_POINT ( 'NONE', #7038 ) ;
#15381=CARTESIAN_POINT ( 'NONE',  ( 5.441664396738000065, -79.05162331913099649, -8.019902302782998760 ) ) ;
#15407=PRESENTATION_STYLE_ASSIGNMENT (( #10990 ) ) ;
#15418=CARTESIAN_POINT ( 'NONE',  ( -5.099999999822000696, -75.20000000017779485, 7.533999751109999828E-10 ) ) ;
#15455=EDGE_CURVE ( 'NONE', #42095, #41372, #9949, .T. ) ;
#15467=CARTESIAN_POINT ( 'NONE',  ( 4.448768332841000372, -79.15906001420199800, 8.980869306721999124 ) ) ;
#15485=CARTESIAN_POINT ( 'NONE',  ( 9.909302118288000116, -78.69441332859899774, 0.1618955519762999840 ) ) ;
#15492=DIRECTION ( 'NONE',  ( 0.000000000000000000, 1.000000000000000000, 0.000000000000000000 ) ) ;
#15512=CARTESIAN_POINT ( 'NONE',  ( 5.684029094576000141, -79.80575194988499277, -7.680196531179999120 ) ) ;
#15516=CARTESIAN_POINT ( 'NONE',  ( 3.595196526684544924, -79.64062500096297015, -8.672428006415348278 ) ) ;
#15531=CARTESIAN_POINT ( 'NONE',  ( 1.529360311630938885, -79.26210760543997935, 9.376159717299817231 ) ) ;
#15548=CARTESIAN_POINT ( 'NONE',  ( 4.871830346738000195, -77.67463667140098948, -8.179061320855998574 ) ) ;
#15556=EDGE_CURVE ( 'NONE', #1911, #5139, #25252, .T. ) ;
#15618=CARTESIAN_POINT ( 'NONE',  ( 8.300970689365454902, -78.10833333333330586, -4.784380313523529438 ) ) ;
#15622=CARTESIAN_POINT ( 'NONE',  ( 2.486604901413133728, -78.75416666666667709, 9.252740428349007118 ) ) ;
#15656=EDGE_CURVE ( 'NONE', #21408, #41593, #25664, .T. ) ;
#15664=VERTEX_POINT ( 'NONE', #32210 ) ;
#15733=CONICAL_SURFACE ( 'NONE', #23274, 5.599999999950999729, 0.2449786631268792425 ) ;
#15737=VERTEX_POINT ( 'NONE', #53393 ) ;
#15740=EDGE_LOOP ( 'NONE', ( #45454, #4108, #3404, #43780 ) ) ;
#15751=CARTESIAN_POINT ( 'NONE',  ( -5.548464554217999556, -78.77021332859899871, -8.076689350464999251 ) ) ;
#15770=CIRCLE ( 'NONE', #26127, 9.199999999999999289 ) ;
#15772=CARTESIAN_POINT ( 'NONE',  ( -3.255457669676000254, -78.10493667140100627, -9.242313942619999168 ) ) ;
#15803=CARTESIAN_POINT ( 'NONE',  ( 8.395992668097999712, -79.41965194988499377, 4.560928606276999808 ) ) ;
#15808=CARTESIAN_POINT ( 'NONE',  ( 9.500000000000000000, -77.14999999999999147, 0.000000000000000000 ) ) ;
#15822=CARTESIAN_POINT ( 'NONE',  ( 8.491818810844479870, -79.18689644516919657, 4.277273810732789450 ) ) ;
#15841=CARTESIAN_POINT ( 'NONE',  ( -9.517358746150001991, -77.50498667140099940, 0.2272806389514000214 ) ) ;
#15843=CYLINDRICAL_SURFACE ( 'NONE', #50673, 9.500000000000000000 ) ;
#15856=CARTESIAN_POINT ( 'NONE',  ( 8.300970689365442468, -78.19166666666667709, 4.784380313523563188 ) ) ;
#15902=CARTESIAN_POINT ( 'NONE',  ( 9.347227379752075294, -78.32137913613844660, 2.683805748252192203 ) ) ;
#15909=CARTESIAN_POINT ( 'NONE',  ( -9.499653450934914645, -79.30027302004205580, 1.387647615217423080E-06 ) ) ;
#15910=CARTESIAN_POINT ( 'NONE',  ( -8.300970689365447797, -77.94166666666667709, -4.784380313523547201 ) ) ;
#15921=DIRECTION ( 'NONE',  ( 0.000000000000000000, -1.000000000000000000, 0.000000000000000000 ) ) ;
#15985=CARTESIAN_POINT ( 'NONE',  ( 5.285146527633999725, -77.77108832859899223, 7.886954000319999381 ) ) ;
#15986=SURFACE_STYLE_FILL_AREA ( #43152 ) ;
#15995=EDGE_CURVE ( 'NONE', #2820, #35308, #10217, .T. ) ;
#16015=DIRECTION ( 'NONE',  ( 1.000000000000000000, 0.000000000000000000, 0.000000000000000000 ) ) ;
#16046=CARTESIAN_POINT ( 'NONE',  ( 4.582566119076999733, -78.09363667140100063, 8.787281441338999244 ) ) ;
#16065=CARTESIAN_POINT ( 'NONE',  ( -7.589275504201999922, -78.06138667140099585, -6.198488971763000066 ) ) ;
#16072=CARTESIAN_POINT ( 'NONE',  ( 1.000000000000000000, -75.20000000000000284, -7.200000000000000178 ) ) ;
#16077=DIRECTION ( 'NONE',  ( -1.000000000000000000, 0.000000000000000000, 0.000000000000000000 ) ) ;
#16097=CARTESIAN_POINT ( 'NONE',  ( 5.896171905175000560, -77.96999999999999886, 7.127247495676000355 ) ) ;
#16116=CARTESIAN_POINT ( 'NONE',  ( 5.732671476984768866, -79.22339475712911394, 7.582784944364554747 ) ) ;
#16124=LINE ( 'NONE', #49673, #28387 ) ;
#16138=CARTESIAN_POINT ( 'NONE',  ( -2.486604901413195456, -77.19583333333333997, 9.252740428348991131 ) ) ;
#16182=EDGE_CURVE ( 'NONE', #42830, #40288, #57326, .T. ) ;
#16190=AXIS2_PLACEMENT_3D ( 'NONE', #55250, #50838, #12119 ) ;
#16197=CARTESIAN_POINT ( 'NONE',  ( 3.350976038670510970, -79.20354908895222934, -8.646094610806894565 ) ) ;
#16238=EDGE_CURVE ( 'NONE', #41814, #23790, #48856, .T. ) ;
#16252=ORIENTED_EDGE ( 'NONE', *, *, #49181, .F. ) ;
#16268=ORIENTED_EDGE ( 'NONE', *, *, #42939, .T. ) ;
#16298=CARTESIAN_POINT ( 'NONE',  ( 4.598371993787000456, -78.79425194988499470, -8.567308531191999421 ) ) ;
#16304=VECTOR ( 'NONE', #5892, 1000.000000000000000 ) ;
#16329=( NAMED_UNIT ( * ) SI_UNIT ( $, .STERADIAN. ) SOLID_ANGLE_UNIT ( ) );
#16336=VERTEX_POINT ( 'NONE', #32847 ) ;
#16342=CARTESIAN_POINT ( 'NONE',  ( -7.544159220956999867, -79.31303667140099378, -6.426939800899999611 ) ) ;
#16351=DIRECTION ( 'NONE',  ( 0.000000000000000000, 1.000000000000000000, -1.243449787580000135E-13 ) ) ;
#16357=CARTESIAN_POINT ( 'NONE',  ( 6.607804308078000233, -79.12991332859898819, -6.725089593472000082 ) ) ;
#16387=CARTESIAN_POINT ( 'NONE',  ( 0.000000000000000000, -78.79999999980499581, 0.000000000000000000 ) ) ;
#16392=CARTESIAN_POINT ( 'NONE',  ( -8.300970689365472666, -78.75833333333335418, 4.784380313523514339 ) ) ;
#16395=ORIENTED_EDGE ( 'NONE', *, *, #15556, .T. ) ;
#16405=CARTESIAN_POINT ( 'NONE',  ( 7.762291303765522343, -79.19863279546440538, 5.476889886169479915 ) ) ;
#16414=CLOSED_SHELL ( 'NONE', ( #35860, #10041, #49518, #53924, #30087, #49142, #20509, #11817, #57174, #43696, #3778, #49788, #23462, #52452, #40848, #12379, #56369, #30777, #54652, #7517, #53597, #47928, #53402, #12953, #29665, #18163, #50780, #56460, #32899, #52127, #42329, #36052, #3802, #29457, #1386, #23445, #48871, #53408, #601, #1991, #35725, #33882, #22477, #32803, #18515, #58351, #50703, #14843, #22707, #37739, #47167, #51314, #51617, #35455, #5517, #31528, #19845, #37031, #24678, #30337 ) ) ;
#16424=CARTESIAN_POINT ( 'NONE',  ( -4.404426062549000598, -77.42016167140099014, 8.439952905775999881 ) ) ;
#16436=CARTESIAN_POINT ( 'NONE',  ( 9.252740428348992907, -78.17083333333334849, 2.486604901413179025 ) ) ;
#16468=ORIENTED_EDGE ( 'NONE', *, *, #47801, .T. ) ;
#16476=VERTEX_POINT ( 'NONE', #34566 ) ;
#16484=CARTESIAN_POINT ( 'NONE',  ( -3.340139707862435969, -78.45202913613843521, 9.133287453676040002 ) ) ;
#16531=CARTESIAN_POINT ( 'NONE',  ( 2.858407197969000002, -77.00000000000000000, 8.797272775729998884 ) ) ;
#16542=CARTESIAN_POINT ( 'NONE',  ( 1.529609450199000076, -77.05228084965399660, 9.371081266747001592 ) ) ;
#16546=DIRECTION ( 'NONE',  ( -1.000000000000000000, 0.000000000000000000, 0.000000000000000000 ) ) ;
#16568=FILL_AREA_STYLE_COLOUR ( '', #20404 ) ;
#16578=CARTESIAN_POINT ( 'NONE',  ( 2.210712544800999879, -79.27330194988499557, -9.468498208576999531 ) ) ;
#16611=CARTESIAN_POINT ( 'NONE',  ( 0.000000000000000000, -75.00000000000000000, 7.200000000000000178 ) ) ;
#16615=ORIENTED_EDGE ( 'NONE', *, *, #44273, .F. ) ;
#16623=CARTESIAN_POINT ( 'NONE',  ( 5.381001269034999979, -79.42917000473400435, -7.930497238065998822 ) ) ;
#16649=CARTESIAN_POINT ( 'NONE',  ( 9.252740428349003565, -79.02916666666671119, -2.486604901413146607 ) ) ;
#16670=DIRECTION ( 'NONE',  ( 1.000000000000000000, 0.000000000000000000, 0.000000000000000000 ) ) ;
#16677=CARTESIAN_POINT ( 'NONE',  ( 2.769824414688999870, -79.21914805011499539, -8.825563591736999669 ) ) ;
#16683=CARTESIAN_POINT ( 'NONE',  ( 9.252740428348991131, -78.57083333333333997, 2.486604901413179913 ) ) ;
#16689=AXIS2_PLACEMENT_3D ( 'NONE', #1918, #19912, #47375 ) ;
#16691=EDGE_CURVE ( 'NONE', #16476, #8049, #44353, .T. ) ;
#16696=CARTESIAN_POINT ( 'NONE',  ( -5.070101917245042777, -79.31948482625490726, 8.043791529919085193 ) ) ;
#16699=AXIS2_PLACEMENT_3D ( 'NONE', #34805, #21527, #39535 ) ;
#16713=EDGE_CURVE ( 'NONE', #9880, #35206, #45352, .T. ) ;
#16724=EDGE_CURVE ( 'NONE', #41331, #31756, #16920, .T. ) ;
#16734=CARTESIAN_POINT ( 'NONE',  ( -9.500000000000000000, -78.39999999999999147, 0.000000000000000000 ) ) ;
#16754=ORIENTED_EDGE ( 'NONE', *, *, #49181, .T. ) ;
#16832=CARTESIAN_POINT ( 'NONE',  ( -2.205007487985999770, -77.08380584965398441, 9.235565851336001941 ) ) ;
#16851=DIRECTION ( 'NONE',  ( 0.000000000000000000, 1.000000000000000000, 0.000000000000000000 ) ) ;
#16867=CIRCLE ( 'NONE', #14036, 9.199999999999999289 ) ;
#16869=CARTESIAN_POINT ( 'NONE',  ( -8.918806285220000518, -78.15755584965400260, 3.872830773119999570 ) ) ;
#16905=ORIENTED_EDGE ( 'NONE', *, *, #1527, .F. ) ;
#16907=ORIENTED_EDGE ( 'NONE', *, *, #54145, .F. ) ;
#16913=CARTESIAN_POINT ( 'NONE',  ( -5.708830652390999738, -78.18073667140099303, 8.101181774151999804 ) ) ;
#16920=LINE ( 'NONE', #26617, #26244 ) ;
#16935=CARTESIAN_POINT ( 'NONE',  ( -7.483407197968000801, -77.00000000000000000, 5.437013583706000297 ) ) ;
#16937=CARTESIAN_POINT ( 'NONE',  ( -5.838193839761688153, -78.87291666666669698, -7.596835002782716728 ) ) ;
#16961=CARTESIAN_POINT ( 'NONE',  ( 8.395992668097999712, -79.29944415034599103, 4.560928606276999808 ) ) ;
#16973=EDGE_CURVE ( 'NONE', #52539, #8827, #36950, .T. ) ;
#16982=CARTESIAN_POINT ( 'NONE',  ( -6.834826231162627330, -79.33866059855550645, 6.598048657260681793 ) ) ;
#17031=DIRECTION ( 'NONE',  ( 0.000000000000000000, 1.000000000000000000, 0.000000000000000000 ) ) ;
#17039=EDGE_LOOP ( 'NONE', ( #35255, #38963, #38081, #9578 ) ) ;
#17053=CARTESIAN_POINT ( 'NONE',  ( 4.741624724934583313, -79.58333333332932114, 8.228481283912117306 ) ) ;
#17060=CARTESIAN_POINT ( 'NONE',  ( 6.954721136732000097, -77.50786001420199511, -7.007357181289999737 ) ) ;
#17091=CARTESIAN_POINT ( 'NONE',  ( -9.233730314758000546, -79.77988667140100176, -2.745678512080999667 ) ) ;
#17098=CARTESIAN_POINT ( 'NONE',  ( -9.500000000000000000, -78.39999999999999147, 0.000000000000000000 ) ) ;
#17100=ORIENTED_EDGE ( 'NONE', *, *, #17294, .F. ) ;
#17112=CARTESIAN_POINT ( 'NONE',  ( 4.897371265365999982, -77.02075584965399457, 7.847181321287999722 ) ) ;
#17145=DIRECTION ( 'NONE',  ( 0.000000000000000000, 0.7071067811866525998, -0.7071067811864425456 ) ) ;
#17148=CARTESIAN_POINT ( 'NONE',  ( 8.384816012895999648, -78.83780194988500511, -4.923277454554000343 ) ) ;
#17154=EDGE_CURVE ( 'NONE', #22005, #8827, #42524, .T. ) ;
#17186=CARTESIAN_POINT ( 'NONE',  ( 6.559997675027998909, -78.44513998579799363, 7.127949055663999722 ) ) ;
#17198=CARTESIAN_POINT ( 'NONE',  ( -8.465317046980235460, -79.43746713076286881, -4.311381249254191417 ) ) ;
#17218=ORIENTED_EDGE ( 'NONE', *, *, #30468, .T. ) ;
#17225=CARTESIAN_POINT ( 'NONE',  ( -4.784380313523538319, -77.38333333333332575, -8.300970689365453126 ) ) ;
#17233=EDGE_CURVE ( 'NONE', #49594, #37512, #56726, .T. ) ;
#17234=B_SPLINE_SURFACE_WITH_KNOTS ( 'NONE', 3, 3, ( 
 ( #50996, #9664, #10544, #14954, #28231, #5234, #50707, #51289, #14658, #46283, #55114, #23525, #55408, #24112, #33247, #55706, #5807, #4943, #9960, #23814, #23239, #45400, #41833, #1695, #37389, #27653, #28528, #46577, #40958, #10844, #45989, #19107, #54827, #549, #18526 ),
 ( #36518, #14368, #50410, #27941, #1119, #37098, #2846, #15548, #52154, #43579, #11140, #2278, #3142, #15841, #33829, #56865, #16424, #51867, #11421, #35566, #21994, #58315, #13426, #21424, #57720, #39714, #31428, #4592, #7847, #25847, #51144, #52582, #57003, #21274, #39282 ),
 ( #57292, #15985, #33975, #49018, #54036, #26854, #49312, #22435, #39852, #8862, #36307, #44885, #31566, #13575, #36011, #31866, #4734, #53742, #49908, #9743, #40743, #17725, #18610, #54332, #40450, #8564, #45184, #35713, #27441, #4435, #13872, #53439, #26554, #49615, #42 ),
 ( #13278, #32156, #9455, #627, #18018, #40147, #45477, #5020, #31270, #9162, #35408, #21845, #12981, #57868, #18316, #22732, #30979, #23024, #41036, #58159, #36598, #27143, #54622, #336, #17421, #14158, #27731, #50195, #45775, #44583, #4140, #22138, #55488, #23891, #32735 ) ),
 .UNSPECIFIED., .F., .F., .F.,
 ( 4, 4 ),
 ( 4, 1, 1, 1, 1, 1, 1, 1, 1, 1, 1, 1, 1, 1, 1, 1, 1, 1, 1, 1, 1, 1, 1, 1, 1, 1, 1, 1, 1, 1, 1, 1, 4 ),
 ( -0.1377334280162000046, 1.137733428016000081 ),
 ( -0.01298507462686999958, 0.008115671641791000201, 0.02921641791044999811, 0.05031716417909999628, 0.07141791044776001074, 0.09251865671641999744, 0.1136194029850999959, 0.1347201492536999889, 0.1558208955223999992, 0.1769216417910000061, 0.1980223880596999886, 0.2191231343283999988, 0.2402238805970000057, 0.2613246268657000160, 0.2824253731342999951, 0.3035261194030000054, 0.3246268656715999845, 0.3457276119402999948, 0.3668283582090000050, 0.3879291044776000397, 0.4090298507462999944, 0.4301305970149000291, 0.4512313432835999838, 0.4723320895522000185, 0.4934328358209000287, 0.5145335820895999834, 0.5356343283582000181, 0.5567350746268999728, 0.5778358208955000075, 0.5989365671641999622, 0.6200373134327999969, 0.6411380597014999516, 0.6622388059702000174 ),
 .UNSPECIFIED. ) ;
#17260=CARTESIAN_POINT ( 'NONE',  ( -4.205654323444776743, -79.31107025363671426, 8.523780649771993012 ) ) ;
#17294=EDGE_CURVE ( 'NONE', #51311, #22854, #48172, .T. ) ;
#17320=ORIENTED_EDGE ( 'NONE', *, *, #31993, .F. ) ;
#17322=ORIENTED_EDGE ( 'NONE', *, *, #56415, .F. ) ;
#17324=CIRCLE ( 'NONE', #10743, 1.000000000000000000 ) ;
#17335=CARTESIAN_POINT ( 'NONE',  ( 7.545211988112344947, -79.56380208332930692, 5.799587082756866963 ) ) ;
#17344=CARTESIAN_POINT ( 'NONE',  ( 5.915537232129000067, -77.08008667140099135, 7.766375951189000482 ) ) ;
#17351=CARTESIAN_POINT ( 'NONE',  ( 8.857115352654000517, -79.36940095943376150, -3.584237475251999872 ) ) ;
#17352=CIRCLE ( 'NONE', #30541, 1.000000000000000000 ) ;
#17398=EDGE_LOOP ( 'NONE', ( #11173, #43551, #35968, #6676, #24777 ) ) ;
#17421=CARTESIAN_POINT ( 'NONE',  ( 6.848349084398000386, -77.06641498579800498, -6.921892615137999805 ) ) ;
#17427=CARTESIAN_POINT ( 'NONE',  ( 0.000000000000000000, -80.70000000003399521, 0.000000000000000000 ) ) ;
#17434=CARTESIAN_POINT ( 'NONE',  ( 4.837913609831387518, -77.00000000000001421, 7.928126058622019023 ) ) ;
#17437=CARTESIAN_POINT ( 'NONE',  ( 9.722066209057999231, -78.88135194988498711, 0.1588365413100999990 ) ) ;
#17441=ORIENTED_EDGE ( 'NONE', *, *, #44862, .F. ) ;
#17442=CARTESIAN_POINT ( 'NONE',  ( -2.370458031814262512, -78.19500000000000739, 9.242975026304344865 ) ) ;
#17454=EDGE_LOOP ( 'NONE', ( #45741, #40268, #22342, #33451, #42630 ) ) ;
#17470=ORIENTED_EDGE ( 'NONE', *, *, #19177, .T. ) ;
#17471=CARTESIAN_POINT ( 'NONE',  ( 8.300970689365454902, -78.60833333333327744, -4.784380313523529438 ) ) ;
#17472=CARTESIAN_POINT ( 'NONE',  ( 9.652542402417001455, -76.94351332859899628, 0.04854625845423999470 ) ) ;
#17480=CARTESIAN_POINT ( 'NONE',  ( -7.374059913654000376, -79.18548998579800013, -6.282030610069000431 ) ) ;
#17484=ORIENTED_EDGE ( 'NONE', *, *, #14549, .F. ) ;
#17488=CARTESIAN_POINT ( 'NONE',  ( 9.500000000000000000, -77.64999999999999147, 0.000000000000000000 ) ) ;
#17491=CARTESIAN_POINT ( 'NONE',  ( -6.781111407274376113, -79.46151114110770664, -6.653164290666497394 ) ) ;
#17514=AXIS2_PLACEMENT_3D ( 'NONE', #55351, #37040, #32304 ) ;
#17548=ORIENTED_EDGE ( 'NONE', *, *, #40614, .F. ) ;
#17556=CARTESIAN_POINT ( 'NONE',  ( -5.569985714943742394, -79.32475174562625853, 7.695716824889310637 ) ) ;
#17594=CARTESIAN_POINT ( 'NONE',  ( 7.565372432932000457, -79.70598667140099280, -5.616098813059000605 ) ) ;
#17611=ORIENTED_EDGE ( 'NONE', *, *, #41867, .T. ) ;
#17627=ORIENTED_EDGE ( 'NONE', *, *, #9369, .T. ) ;
#17641=CARTESIAN_POINT ( 'NONE',  ( 9.334420024193999410, -77.54426001420199555, -3.215556494258000164 ) ) ;
#17670=CARTESIAN_POINT ( 'NONE',  ( 0.000000000000000000, -80.79999999999999716, 0.000000000000000000 ) ) ;
#17679=CARTESIAN_POINT ( 'NONE',  ( -3.992191694170000194, -79.72926001420199782, 8.886347659747999117 ) ) ;
#17688=AXIS2_PLACEMENT_3D ( 'NONE', #22802, #54683, #49977 ) ;
#17725=CARTESIAN_POINT ( 'NONE',  ( 9.266295309513999712, -77.21501332859899946, 2.616508480087999633 ) ) ;
#17736=CARTESIAN_POINT ( 'NONE',  ( 6.184758847501745649, -77.00000000000000000, 6.951421119677088534 ) ) ;
#17739=CARTESIAN_POINT ( 'NONE',  ( 4.495978696100999983, -77.90669805011499705, 8.621246072682998474 ) ) ;
#17780=CARTESIAN_POINT ( 'NONE',  ( -5.644471715163000169, -78.11696332859899883, 8.009852484315999277 ) ) ;
#17794=CARTESIAN_POINT ( 'NONE',  ( -8.817229174565222038, -79.43036102351236138, -3.552007249728367455 ) ) ;
#17811=CARTESIAN_POINT ( 'NONE',  ( -9.499999999999998224, -78.31041666666665435, -1.243547092045960367 ) ) ;
#17816=CARTESIAN_POINT ( 'NONE',  ( -5.148784662568076406E-06, -79.56241750339395935, -9.437165819784945953 ) ) ;
#17826=EDGE_CURVE ( 'NONE', #1911, #15146, #31067, .T. ) ;
#17848=ORIENTED_EDGE ( 'NONE', *, *, #887, .F. ) ;
#17859=CARTESIAN_POINT ( 'NONE',  ( -1.760571071064350956, -79.28971201036856087, 9.336322274714841996 ) ) ;
#17864=ORIENTED_EDGE ( 'NONE', *, *, #43250, .T. ) ;
#17875=CARTESIAN_POINT ( 'NONE',  ( 4.834410198815040971, -77.71759693750338727, -8.116238590442467427 ) ) ;
#17895=MANIFOLD_SOLID_BREP ( 'Stock-MAS-694-1', #16414 ) ;
#17896=CARTESIAN_POINT ( 'NONE',  ( 6.529408856002000050, -79.19118667140099888, -7.077026392590000548 ) ) ;
#17919=EDGE_LOOP ( 'NONE', ( #2320, #16905, #39657, #41606 ) ) ;
#17941=CARTESIAN_POINT ( 'NONE',  ( -1.311199674450999941, -77.43506001420199425, -9.785292850414998966 ) ) ;
#17999=CARTESIAN_POINT ( 'NONE',  ( -7.264520526674999701, -77.62562305011499575, -6.114261184555999762 ) ) ;
#18018=CARTESIAN_POINT ( 'NONE',  ( 9.732069852918000308, -77.63191498579799088, 0.3150258461668000165 ) ) ;
#18028=CARTESIAN_POINT ( 'NONE',  ( 5.100000000000000533, -76.79999999999999716, 0.000000000000000000 ) ) ;
#18031=CARTESIAN_POINT ( 'NONE',  ( -9.631455446501000495, -78.02079415034600629, -1.333735528292999906 ) ) ;
#18049=ORIENTED_EDGE ( 'NONE', *, *, #27832, .T. ) ;
#18075=CARTESIAN_POINT ( 'NONE',  ( 6.458817137649000450, -79.31613998579798874, -6.573457973844999636 ) ) ;
#18076=CYLINDRICAL_SURFACE ( 'NONE', #18137, 5.100000000000000533 ) ;
#18084=CARTESIAN_POINT ( 'NONE',  ( 8.300970689365454902, -77.60833333333330586, -4.784380313523529438 ) ) ;
#18089=CARTESIAN_POINT ( 'NONE',  ( -4.966864318370061149, -79.48090711910747075, -8.097943653986082069 ) ) ;
#18096=ORIENTED_EDGE ( 'NONE', *, *, #28451, .F. ) ;
#18108=CARTESIAN_POINT ( 'NONE',  ( 9.500000000000005329, -78.53958333333333997, -1.243547092045939939 ) ) ;
#18137=AXIS2_PLACEMENT_3D ( 'NONE', #35771, #26910, #45828 ) ;
#18156=CARTESIAN_POINT ( 'NONE',  ( -9.470942015330143349, -79.39363629237638520, 0.7411628763851737522 ) ) ;
#18163=ADVANCED_FACE ( 'NONE', ( #26143 ), #35459, .T. ) ;
#18193=CARTESIAN_POINT ( 'NONE',  ( 4.052275399702000236, -79.23156001420198891, -8.386988472880998913 ) ) ;
#18206=CARTESIAN_POINT ( 'NONE',  ( 0.000000000000000000, -78.79999999980499581, 0.000000000000000000 ) ) ;
#18244=CARTESIAN_POINT ( 'NONE',  ( 1.898691536689999904, -77.18026001420200544, 9.688454896930000615 ) ) ;
#18256=LINE ( 'NONE', #40978, #25163 ) ;
#18295=CARTESIAN_POINT ( 'NONE',  ( 8.503129636637000388, -77.84335194988499040, -4.225430575863000193 ) ) ;
#18316=CARTESIAN_POINT ( 'NONE',  ( -9.045487252274998724, -77.34916498579799793, 3.604392171359999786 ) ) ;
#18325=CARTESIAN_POINT ( 'NONE',  ( 9.290488860786039638, -77.00000000000002842, -1.721794440864784059 ) ) ;
#18327=CARTESIAN_POINT ( 'NONE',  ( 9.722066209057999231, -78.76114415034598437, 0.1588365413100999990 ) ) ;
#18365=CARTESIAN_POINT ( 'NONE',  ( -0.5292728922702000238, -78.74998998579799547, -9.672698560386999489 ) ) ;
#18393=CYLINDRICAL_SURFACE ( 'NONE', #25899, 1.000000000000000000 ) ;
#18405=CARTESIAN_POINT ( 'NONE',  ( 5.896171905175000560, -77.96999999999999886, 7.127247495676000355 ) ) ;
#18409=CARTESIAN_POINT ( 'NONE',  ( -9.252740428348994683, -77.32083333333332575, -2.486604901413163926 ) ) ;
#18472=VERTEX_POINT ( 'NONE', #46809 ) ;
#18497=ORIENTED_EDGE ( 'NONE', *, *, #17826, .F. ) ;
#18498=DIRECTION ( 'NONE',  ( 1.000000000000000000, 0.000000000000000000, 0.000000000000000000 ) ) ;
#18515=ADVANCED_FACE ( 'NONE', ( #55940 ), #38207, .T. ) ;
#18526=CARTESIAN_POINT ( 'NONE',  ( -6.103045505686000460, -77.00326001420198452, 6.905034692672999519 ) ) ;
#18533=CARTESIAN_POINT ( 'NONE',  ( -0.1212951196120999886, -77.81711332859900665, -9.651867515931000341 ) ) ;
#18589=CARTESIAN_POINT ( 'NONE',  ( -5.597970637881999778, -77.05522694988499666, 7.669424558767000022 ) ) ;
#18590=CIRCLE ( 'NONE', #16689, 11.65000000000000036 ) ;
#18603=CIRCLE ( 'NONE', #51613, 1.199999999999999956 ) ;
#18610=CARTESIAN_POINT ( 'NONE',  ( 9.597740827301000976, -77.18673832859900585, -0.7705299494857000830 ) ) ;
#18618=CARTESIAN_POINT ( 'NONE',  ( 7.665367164120238996, -77.00000000000001421, 5.330550266068665444 ) ) ;
#18694=CARTESIAN_POINT ( 'NONE',  ( -9.204193785523999694, -77.16974903538300623, -2.332437886131999871 ) ) ;
#18703=DIRECTION ( 'NONE',  ( 0.000000000000000000, -1.000000000000000000, 0.000000000000000000 ) ) ;
#18719=DIRECTION ( 'NONE',  ( 1.000000000000000000, 0.000000000000000000, 0.000000000000000000 ) ) ;
#18739=EDGE_CURVE ( 'NONE', #8049, #8827, #20613, .T. ) ;
#18750=CARTESIAN_POINT ( 'NONE',  ( 8.353603324983998490, -78.77841001420199518, -4.904950430745999235 ) ) ;
#18768=CARTESIAN_POINT ( 'NONE',  ( 9.832881223348001853, -79.13383998579799083, 0.5566273142183999489 ) ) ;
#18792=ORIENTED_EDGE ( 'NONE', *, *, #40129, .F. ) ;
#18799=VERTEX_POINT ( 'NONE', #56516 ) ;
#18801=CARTESIAN_POINT ( 'NONE',  ( 9.064091738852273039, -79.17377439753506962, 2.844017911560304146 ) ) ;
#18822=CARTESIAN_POINT ( 'NONE',  ( -6.374294731314999574, -77.12551332859899844, 7.248560140069000290 ) ) ;
#18829=DIRECTION ( 'NONE',  ( 0.000000000000000000, -1.000000000000000000, 0.000000000000000000 ) ) ;
#18852=CARTESIAN_POINT ( 'NONE',  ( -6.187990949381768857, -77.00000000000000000, 6.880426350252046852 ) ) ;
#18856=CARTESIAN_POINT ( 'NONE',  ( 9.342273945276998504, -79.45871332859898928, 1.855243057797000050 ) ) ;
#18866=EDGE_LOOP ( 'NONE', ( #5213, #31276, #32408, #14583, #18920, #5285, #44617, #16615, #47391 ) ) ;
#18875=CARTESIAN_POINT ( 'NONE',  ( -2.205007487985999770, -76.96359805011501010, 9.235565851336001941 ) ) ;
#18882=CARTESIAN_POINT ( 'NONE',  ( -9.252740428349008894, -77.77916666666668277, 2.486604901413127955 ) ) ;
#18909=ORIENTED_EDGE ( 'NONE', *, *, #53369, .T. ) ;
#18912=CONICAL_SURFACE ( 'NONE', #51922, 11.54999999996000071, 0.7853981633972997312 ) ;
#18920=ORIENTED_EDGE ( 'NONE', *, *, #29687, .F. ) ;
#18929=AXIS2_PLACEMENT_3D ( 'NONE', #12815, #39111, #8107 ) ;
#18930=CARTESIAN_POINT ( 'NONE',  ( -9.329078564973897869, -76.99999999999998579, -0.4380577504101695885 ) ) ;
#18933=AXIS2_PLACEMENT_3D ( 'NONE', #25147, #7721, #38435 ) ;
#18937=CARTESIAN_POINT ( 'NONE',  ( -8.084188863228343180, -79.71354166666438346, -4.672135182878759174 ) ) ;
#18940=CARTESIAN_POINT ( 'NONE',  ( -9.500000000000007105, -77.89249999999998408, 0.8953539062730669906 ) ) ;
#18992=CARTESIAN_POINT ( 'NONE',  ( 7.483407197968000801, -79.75000000000000000, -5.437013583705000208 ) ) ;
#18997=CONICAL_SURFACE ( 'NONE', #21794, 9.099999999966000175, 0.7853981633972997312 ) ;
#19005=CARTESIAN_POINT ( 'NONE',  ( 5.838193839761705917, -77.97708333333333997, -7.596835002782701629 ) ) ;
#19024=CARTESIAN_POINT ( 'NONE',  ( -9.144741847372999999, -78.85421001420199616, -4.101371784086000005 ) ) ;
#19064=CARTESIAN_POINT ( 'NONE',  ( 2.823168074518000115, -79.09231332859899055, -8.995533882827999150 ) ) ;
#19079=AXIS2_PLACEMENT_3D ( 'NONE', #24069, #51831, #20803 ) ;
#19080=ORIENTED_EDGE ( 'NONE', *, *, #40129, .T. ) ;
#19084=DIRECTION ( 'NONE',  ( 0.000000000000000000, 1.000000000000000000, 0.000000000000000000 ) ) ;
#19107=CARTESIAN_POINT ( 'NONE',  ( -9.324187677468000146, -77.05981001420200016, 1.279235053889000051 ) ) ;
#19146=CARTESIAN_POINT ( 'NONE',  ( -7.504986677982999232, -79.68093998579799120, -5.686679248032999290 ) ) ;
#19167=CARTESIAN_POINT ( 'NONE',  ( 6.214091009702999102, -77.81182694988498838, -7.179311535719000048 ) ) ;
#19172=EDGE_CURVE ( 'NONE', #13771, #2820, #347, .T. ) ;
#19177=EDGE_CURVE ( 'NONE', #4309, #43096, #53425, .T. ) ;
#19222=EDGE_CURVE ( 'NONE', #18472, #15737, #18256, .T. ) ;
#19228=ORIENTED_EDGE ( 'NONE', *, *, #20290, .F. ) ;
#19230=CARTESIAN_POINT ( 'NONE',  ( -7.541360678298866027, -77.84749999999998238, 5.846326858574209417 ) ) ;
#19269=CARTESIAN_POINT ( 'NONE',  ( 2.210712544800999879, -79.33340584965399955, -9.468498208576999531 ) ) ;
#19297=CARTESIAN_POINT ( 'NONE',  ( -2.486604901413152824, -77.90416666666666856, -9.252740428349003565 ) ) ;
#19318=CARTESIAN_POINT ( 'NONE',  ( -9.500000000000000000, -77.89999999999999147, 0.000000000000000000 ) ) ;
#19320=ORIENTED_EDGE ( 'NONE', *, *, #42418, .T. ) ;
#19334=CARTESIAN_POINT ( 'NONE',  ( -3.327183877592000183, -78.47356001420199334, 9.097860994781999722 ) ) ;
#19353=CARTESIAN_POINT ( 'NONE',  ( 5.793497013506000215, -79.61881332859898919, -7.828108358733000038 ) ) ;
#19362=CARTESIAN_POINT ( 'NONE',  ( -6.053394164830000257, -79.64034805011499429, -7.392643757108000813 ) ) ;
#19372=CARTESIAN_POINT ( 'NONE',  ( 9.199999999999999289, -77.00000000000000000, 0.000000000000000000 ) ) ;
#19388=DIRECTION ( 'NONE',  ( 0.7071067811865470176, -0.7071067811865470176, 3.647649194621239524E-08 ) ) ;
#19401=CARTESIAN_POINT ( 'NONE',  ( -8.300970689365472666, -77.25833333333336839, 4.784380313523514339 ) ) ;
#19406=CARTESIAN_POINT ( 'NONE',  ( 9.500000000000000000, -77.14999999999999147, 0.000000000000000000 ) ) ;
#19415=CARTESIAN_POINT ( 'NONE',  ( -5.505695391233000002, -78.58694415034598535, -8.014431902511001127 ) ) ;
#19420=CARTESIAN_POINT ( 'NONE',  ( 5.099999999822000696, -75.20000000017779485, -7.534001399281000208E-10 ) ) ;
#19422=ORIENTED_EDGE ( 'NONE', *, *, #21590, .F. ) ;
#19464=ORIENTED_EDGE ( 'NONE', *, *, #35611, .T. ) ;
#19477=EDGE_LOOP ( 'NONE', ( #13104, #20962, #16395 ) ) ;
#19509=CARTESIAN_POINT ( 'NONE',  ( -9.320350064846081750, -77.00000000000000000, 0.5764697903331228446 ) ) ;
#19513=CIRCLE ( 'NONE', #52506, 1.000000000000000000 ) ;
#19525=CARTESIAN_POINT ( 'NONE',  ( -8.914528142879424522, -79.37164879542098106, 3.287790175345898902 ) ) ;
#19530=ORIENTED_EDGE ( 'NONE', *, *, #43250, .F. ) ;
#19581=ORIENTED_EDGE ( 'NONE', *, *, #32809, .F. ) ;
#19620=CARTESIAN_POINT ( 'NONE',  ( -5.580112777935000601, -77.99451001420200669, 7.918523194479999638 ) ) ;
#19641=CARTESIAN_POINT ( 'NONE',  ( 2.791340874175999520, -79.15608667140098476, -8.894122046368000412 ) ) ;
#19649=CARTESIAN_POINT ( 'NONE',  ( 8.857115352654000517, -79.40955584965399794, -3.584237475251999872 ) ) ;
#19650=FACE_OUTER_BOUND ( 'NONE', #51340, .T. ) ;
#19669=CARTESIAN_POINT ( 'NONE',  ( 6.101084436648303466, -79.21938963383225030, 7.282006857732869598 ) ) ;
#19706=CARTESIAN_POINT ( 'NONE',  ( 2.210712544800999879, -79.15309415034599283, -9.468498208576999531 ) ) ;
#19756=CARTESIAN_POINT ( 'NONE',  ( 2.013948389145618467, -78.19072913613844378, -9.514067696212755720 ) ) ;
#19806=CARTESIAN_POINT ( 'NONE',  ( -8.033785430678635819, -76.99999999999998579, -4.895566815014301909 ) ) ;
#19813=CARTESIAN_POINT ( 'NONE',  ( -6.234243430155317789, -79.72916666666543506, -6.929937226105533199 ) ) ;
#19841=CARTESIAN_POINT ( 'NONE',  ( -0.9999999970759999579, -75.20000000292399989, -7.200000017194999380 ) ) ;
#19845=ADVANCED_FACE ( 'NONE', ( #6098, #41829 ), #32652, .T. ) ;
#19853=CARTESIAN_POINT ( 'NONE',  ( -0.8481231068849000021, -79.07210584965399391, 9.686304223355000076 ) ) ;
#19859=ORIENTED_EDGE ( 'NONE', *, *, #3816, .T. ) ;
#19873=AXIS2_PLACEMENT_3D ( 'NONE', #35663, #26230, #43965 ) ;
#19882=CARTESIAN_POINT ( 'NONE',  ( 1.243547092045970581, -77.93541666666665435, -9.500000000000000000 ) ) ;
#19900=CARTESIAN_POINT ( 'NONE',  ( 1.958352037450999727, -78.68001001420199714, 9.829161269560000136 ) ) ;
#19912=DIRECTION ( 'NONE',  ( 0.000000000000000000, 1.000000000000000000, 0.000000000000000000 ) ) ;
#19920=CARTESIAN_POINT ( 'NONE',  ( 2.253288347564000205, -79.08636332859900619, -9.650850687256999905 ) ) ;
#19927=FACE_OUTER_BOUND ( 'NONE', #10600, .T. ) ;
#19940=CARTESIAN_POINT ( 'NONE',  ( 8.654165682147999306, -79.16893998579799074, 4.701175118119000018 ) ) ;
#19941=CARTESIAN_POINT ( 'NONE',  ( -9.500000000000000000, -77.39999999999999147, 0.000000000000000000 ) ) ;
#19945=CARTESIAN_POINT ( 'NONE',  ( 5.100000000000000533, -75.20000000000000284, 0.000000000000000000 ) ) ;
#19950=CARTESIAN_POINT ( 'NONE',  ( -8.630067035710000667, -79.66535194988499313, -4.100810385846999750 ) ) ;
#19965=ORIENTED_EDGE ( 'NONE', *, *, #22057, .T. ) ;
#19971=CARTESIAN_POINT ( 'NONE',  ( 8.972094814454390388, -79.17629006715765172, 3.124824076624122871 ) ) ;
#20046=ORIENTED_EDGE ( 'NONE', *, *, #47736, .T. ) ;
#20051=CARTESIAN_POINT ( 'NONE',  ( 4.001451577097999923, -77.84924415034599576, 8.339717337904000161 ) ) ;
#20062=CARTESIAN_POINT ( 'NONE',  ( -7.596835002782708735, -77.95208333333333428, -5.838193839761694370 ) ) ;
#20107=ORIENTED_EDGE ( 'NONE', *, *, #28451, .T. ) ;
#20109=CARTESIAN_POINT ( 'NONE',  ( -8.872994237323272415, -77.86999999999999034, 3.510218210012938211 ) ) ;
#20113=CARTESIAN_POINT ( 'NONE',  ( -9.438184056264791622, -79.39065464712832920, 1.083930077607391240 ) ) ;
#20147=CARTESIAN_POINT ( 'NONE',  ( 4.598371993787000456, -78.85435584965399869, -8.567308531191999421 ) ) ;
#20191=CARTESIAN_POINT ( 'NONE',  ( -0.8547114690830001082, -79.07506332859900056, 9.761549055228000427 ) ) ;
#20202=CARTESIAN_POINT ( 'NONE',  ( 9.500000000000000000, -77.64999999999999147, 0.000000000000000000 ) ) ;
#20211=CARTESIAN_POINT ( 'NONE',  ( -0.5353773281849999455, -78.62753667140100333, -9.784259853904000437 ) ) ;
#20221=CARTESIAN_POINT ( 'NONE',  ( 3.938171349113054998, -79.24333333333341045, -8.369041066855391620 ) ) ;
#20239=CARTESIAN_POINT ( 'NONE',  ( -9.554796630153999715, -79.69035584965399721, -0.02401403847836000235 ) ) ;
#20243=CARTESIAN_POINT ( 'NONE',  ( 8.300970689365442468, -77.19166666666667709, 4.784380313523563188 ) ) ;
#20257=CARTESIAN_POINT ( 'NONE',  ( 5.194870660562412645, -79.22882422843130712, 7.960803537416587972 ) ) ;
#20286=CARTESIAN_POINT ( 'NONE',  ( 7.596835002782696300, -78.20208333333334849, 5.838193839761711246 ) ) ;
#20290=EDGE_CURVE ( 'NONE', #37723, #89, #25201, .T. ) ;
#20313=CIRCLE ( 'NONE', #34405, 1.000000000000000000 ) ;
#20330=CARTESIAN_POINT ( 'NONE',  ( 4.574312611392000072, -77.34484415034599181, 8.320643751074999983 ) ) ;
#20382=CARTESIAN_POINT ( 'NONE',  ( -9.141390146399626104, -76.99999999999998579, 1.754763298405772165 ) ) ;
#20395=DIRECTION ( 'NONE',  ( 0.000000000000000000, 1.000000000000000000, 0.000000000000000000 ) ) ;
#20404=COLOUR_RGB ( '', 0.31764706, 0.68627451, 0.89019608) ;
#20440=DIRECTION ( 'NONE',  ( 0.000000000000000000, 1.000000000000000000, -1.776356839400000238E-14 ) ) ;
#20478=CARTESIAN_POINT ( 'NONE',  ( -9.676327351641999641, -79.20571332859898916, -1.545051445613999874 ) ) ;
#20480=CARTESIAN_POINT ( 'NONE',  ( 0.000000000000000000, -75.09999999996229292, 0.000000000000000000 ) ) ;
#20488=CARTESIAN_POINT ( 'NONE',  ( -9.431564212231878130, -79.40938065491944542, -1.151173011385696165 ) ) ;
#20497=CARTESIAN_POINT ( 'NONE',  ( -9.042797184480999562, -78.47666332859900251, -4.055650103703999143 ) ) ;
#20502=CARTESIAN_POINT ( 'NONE',  ( 1.243547092045970581, -78.93541666666665435, -9.500000000000000000 ) ) ;
#20509=ADVANCED_FACE ( 'NONE', ( #10012 ), #40328, .F. ) ;
#20523=CARTESIAN_POINT ( 'NONE',  ( -5.505695391232999114, -78.72709514476063930, -8.014431902511001127 ) ) ;
#20526=CARTESIAN_POINT ( 'NONE',  ( 2.769824414688999870, -79.15904415034599140, -8.825563591736999669 ) ) ;
#20529=CONICAL_SURFACE ( 'NONE', #28049, 9.349999999968000353, 0.7853981633972997312 ) ;
#20533=CARTESIAN_POINT ( 'NONE',  ( 9.499999999999998224, -78.56041666666665435, 1.243547092045980129 ) ) ;
#20545=CARTESIAN_POINT ( 'NONE',  ( 9.031152101340357063, -79.17469186335426912, 2.946796958029828772 ) ) ;
#20564=CARTESIAN_POINT ( 'NONE',  ( 1.243547092045928615, -77.16458333333332575, 9.500000000000003553 ) ) ;
#20575=DIRECTION ( 'NONE',  ( 0.000000000000000000, -1.000000000000000000, 0.000000000000000000 ) ) ;
#20585=ORIENTED_EDGE ( 'NONE', *, *, #10925, .F. ) ;
#20596=EDGE_LOOP ( 'NONE', ( #40691, #33774, #27633, #36794, #16268 ) ) ;
#20613=B_SPLINE_CURVE_WITH_KNOTS ( 'NONE', 3,
 ( #43515, #21644, #34634, #3641, #39076, #16937, #39651, #29340, #26066, #20502, #25209, #3076, #7498, #25496, #34054, #16649, #11933, #29911 ),
 .UNSPECIFIED., .F., .F.,
 ( 4, 2, 2, 2, 2, 2, 2, 2, 4 ),
 ( 0.000000000000000000, 0.1250000000000000833, 0.2500000000000001665, 0.3750000000000002220, 0.5000000000000002220, 0.6250000000000002220, 0.7500000000000001110, 0.8750000000000001110, 1.000000000000000000 ),
 .UNSPECIFIED. ) ;
#20616=CARTESIAN_POINT ( 'NONE',  ( 9.136202122873999798, -77.28179415034600197, 2.585973524422000125 ) ) ;
#20619=VECTOR ( 'NONE', #28973, 1000.000000000000114 ) ;
#20628=CARTESIAN_POINT ( 'NONE',  ( -0.1240611623467000046, -77.94466001420200030, -9.871970996624998662 ) ) ;
#20643=AXIS2_PLACEMENT_3D ( 'NONE', #42858, #23960, #41979 ) ;
#20663=CARTESIAN_POINT ( 'NONE',  ( 8.266198729306507786, -79.50520833333278858, -4.776057930729986190 ) ) ;
#20688=DIRECTION ( 'NONE',  ( 0.000000000000000000, 1.000000000000000000, 0.000000000000000000 ) ) ;
#20714=CARTESIAN_POINT ( 'NONE',  ( 5.285315739688693171, -77.00000000000001421, 7.652295706397369557 ) ) ;
#20717=CARTESIAN_POINT ( 'NONE',  ( 6.584508673715999905, -78.44585194988499666, 7.154582167228999978 ) ) ;
#20737=CARTESIAN_POINT ( 'NONE',  ( 4.009346575041191407, -79.10969738753867375, -8.520289397331099579 ) ) ;
#20761=CARTESIAN_POINT ( 'NONE',  ( -9.170454433240001535, -79.22593667140100138, 3.758088286126999744 ) ) ;
#20766=EDGE_LOOP ( 'NONE', ( #29737, #48110, #44713, #7660, #46781 ) ) ;
#20778=CARTESIAN_POINT ( 'NONE',  ( -5.708830652390999738, -77.86696332859899883, 8.101181774151999804 ) ) ;
#20779=DIRECTION ( 'NONE',  ( -1.000000000000000000, 0.000000000000000000, 0.000000000000000000 ) ) ;
#20803=DIRECTION ( 'NONE',  ( 0.000000000000000000, 0.000000000000000000, -1.000000000000000000 ) ) ;
#20825=CARTESIAN_POINT ( 'NONE',  ( 7.446016869863558263, -79.20295307825982434, 5.901058708005812115 ) ) ;
#20830=CARTESIAN_POINT ( 'NONE',  ( -6.053718295315133169, -79.62010282387937821, -7.393039598043110949 ) ) ;
#20894=EDGE_CURVE ( 'NONE', #24677, #31891, #39545, .T. ) ;
#20903=CARTESIAN_POINT ( 'NONE',  ( -8.998590793623751694, -79.01817913613845690, 3.687657890823406337 ) ) ;
#20917=STYLED_ITEM ( 'NONE', ( #22772 ), #1805 ) ;
#20962=ORIENTED_EDGE ( 'NONE', *, *, #29182, .T. ) ;
#21002=CARTESIAN_POINT ( 'NONE',  ( 5.279327442448000340, -79.30233528321798531, -7.780650776298999816 ) ) ;
#21018=CARTESIAN_POINT ( 'NONE',  ( 0.000000000000000000, -75.10000000284179578, 7.200000000000000178 ) ) ;
#21027=CARTESIAN_POINT ( 'NONE',  ( 5.896171905175000560, -77.86999999999999034, 7.127247495676000355 ) ) ;
#21047=CARTESIAN_POINT ( 'NONE',  ( -5.875581754031000692, -79.18238667140099096, 7.981103691720999649 ) ) ;
#21065=CARTESIAN_POINT ( 'NONE',  ( 9.418360348373997937, -78.27913667140100529, 2.704229673158000224 ) ) ;
#21115=CARTESIAN_POINT ( 'NONE',  ( -3.652956595797749895, -79.30607455077640111, 8.769390947670537173 ) ) ;
#21135=EDGE_CURVE ( 'NONE', #37236, #23864, #57052, .T. ) ;
#21143=CARTESIAN_POINT ( 'NONE',  ( 4.784380313523522332, -78.23333333333333428, 8.300970689365462007 ) ) ;
#21196=CARTESIAN_POINT ( 'NONE',  ( 5.838193839761703252, -78.07708333333333428, -7.596835002782702517 ) ) ;
#21200=CARTESIAN_POINT ( 'NONE',  ( 4.784380313523522332, -78.73333333333332007, 8.300970689365462007 ) ) ;
#21231=CARTESIAN_POINT ( 'NONE',  ( 8.185149126674000186, -79.55108667140099499, 5.079755422656999642 ) ) ;
#21239=CARTESIAN_POINT ( 'NONE',  ( -8.561416052707739865, -77.00000000000000000, 3.586226970955711302 ) ) ;
#21250=CARTESIAN_POINT ( 'NONE',  ( -9.454379850511999805, -77.68278084965399444, 0.8787206290761000460 ) ) ;
#21256=DIRECTION ( 'NONE',  ( 0.8090169943750002979, 0.000000000000000000, -0.5877852522924001955 ) ) ;
#21274=CARTESIAN_POINT ( 'NONE',  ( -7.000686966495000441, -76.94891167140099242, 6.253505135046999897 ) ) ;
#21282=DIRECTION ( 'NONE',  ( 0.000000000000000000, -0.9701425001453282126, -0.2425356250363475685 ) ) ;
#21287=CARTESIAN_POINT ( 'NONE',  ( -7.401612602209000968, -79.12609805011500441, -6.305503003149000030 ) ) ;
#21316=DIRECTION ( 'NONE',  ( 0.000000000000000000, -1.000000000000000000, 0.000000000000000000 ) ) ;
#21330=CARTESIAN_POINT ( 'NONE',  ( -0.5414817640998000892, -78.87753667140100333, -9.895821147420001296 ) ) ;
#21337=CARTESIAN_POINT ( 'NONE',  ( 2.486604901413172808, -77.54583333333330586, -9.252740428348992907 ) ) ;
#21369=CARTESIAN_POINT ( 'NONE',  ( -5.299999999999999822, -75.00000000000000000, 0.000000000000000000 ) ) ;
#21382=CARTESIAN_POINT ( 'NONE',  ( -9.554796630153999715, -79.51004415034600470, -0.02401403847836000235 ) ) ;
#21404=CARTESIAN_POINT ( 'NONE',  ( 0.7542767905157096164, -79.26850739209180574, 9.471697596554010445 ) ) ;
#21408=VERTEX_POINT ( 'NONE', #35457 ) ;
#21409=ORIENTED_EDGE ( 'NONE', *, *, #37501, .T. ) ;
#21424=CARTESIAN_POINT ( 'NONE',  ( 8.631763462862000580, -77.22223667140100645, -4.015524064286999817 ) ) ;
#21487=CARTESIAN_POINT ( 'NONE',  ( 8.149610418757999852, -77.55328667140099697, 5.375310761231999912 ) ) ;
#21519=CARTESIAN_POINT ( 'NONE',  ( 6.190793678633999875, -79.50046001420199104, -7.521868196643000992 ) ) ;
#21527=DIRECTION ( 'NONE',  ( 0.000000000000000000, 1.000000000000000000, 0.000000000000000000 ) ) ;
#21540=CARTESIAN_POINT ( 'NONE',  ( 9.426477049435000310, -77.43058084965399246, -1.139727483088999849 ) ) ;
#21559=CARTESIAN_POINT ( 'NONE',  ( -9.500094076791862463, -79.39994338716823563, -4.328536937075411965E-07 ) ) ;
#21579=CARTESIAN_POINT ( 'NONE',  ( -0.8481231068849000021, -78.95189805011500539, 9.686304223355000076 ) ) ;
#21590=EDGE_CURVE ( 'NONE', #51311, #12545, #40926, .T. ) ;
#21618=CARTESIAN_POINT ( 'NONE',  ( 8.188916213828999702, -78.92418998579800871, 5.175217742376999830 ) ) ;
#21630=CARTESIAN_POINT ( 'NONE',  ( -4.588273267446388637, -79.48450841110565079, -8.321223633674817322 ) ) ;
#21644=CARTESIAN_POINT ( 'NONE',  ( -9.499999999999998224, -78.81041666666666856, -1.243547092045960367 ) ) ;
#21650=ORIENTED_EDGE ( 'NONE', *, *, #44862, .T. ) ;
#21658=CARTESIAN_POINT ( 'NONE',  ( -9.199999999999999289, -77.00000000000000000, 0.000000000000000000 ) ) ;
#21669=CARTESIAN_POINT ( 'NONE',  ( -6.053394164830000257, -79.58024415034599031, -7.392643757108000813 ) ) ;
#21689=CARTESIAN_POINT ( 'NONE',  ( -5.670780713235441972, -79.32583130080989520, 7.622161873721389647 ) ) ;
#21771=CARTESIAN_POINT ( 'NONE',  ( -9.021895076917001433, -77.22568667140099308, 3.730351835827999896 ) ) ;
#21794=AXIS2_PLACEMENT_3D ( 'NONE', #45302, #35532, #26969 ) ;
#21824=EDGE_LOOP ( 'NONE', ( #13469, #13992, #674 ) ) ;
#21845=CARTESIAN_POINT ( 'NONE',  ( -7.529844411733000342, -77.43398998579799297, -6.173647680939999383 ) ) ;
#21852=DIRECTION ( 'NONE',  ( 0.000000000000000000, 1.000000000000000000, 0.000000000000000000 ) ) ;
#21854=DIRECTION ( 'NONE',  ( 0.2425356250363094601, 0.9701425001453377606, 4.828652960331188457E-10 ) ) ;
#21858=CARTESIAN_POINT ( 'NONE',  ( 4.495978696100999983, -78.02690584965399978, 8.621246072682998474 ) ) ;
#21899=CARTESIAN_POINT ( 'NONE',  ( -9.595602112029999020, -78.14028998579800600, -1.328770664336999863 ) ) ;
#21908=CARTESIAN_POINT ( 'NONE',  ( -9.500000000000000000, -77.39999999999999147, 0.000000000000000000 ) ) ;
#21960=FACE_OUTER_BOUND ( 'NONE', #38102, .T. ) ;
#21975=CARTESIAN_POINT ( 'NONE',  ( -6.028334951382167795, -79.32967556650831398, 7.344047846277041103 ) ) ;
#21981=CARTESIAN_POINT ( 'NONE',  ( 7.685661446562000343, -79.50000000000000000, -5.583959896778000420 ) ) ;
#21994=CARTESIAN_POINT ( 'NONE',  ( 7.689575839419000580, -77.30706167140100149, 5.612681836884999775 ) ) ;
#22005=VERTEX_POINT ( 'NONE', #45975 ) ;
#22009=CARTESIAN_POINT ( 'NONE',  ( 3.324778437932995434, -79.05333333333332746, -8.934722022349857795 ) ) ;
#22011=CARTESIAN_POINT ( 'NONE',  ( -8.618369191482001312, -79.53576001420199759, 4.042276274071999076 ) ) ;
#22035=ORIENTED_EDGE ( 'NONE', *, *, #16973, .T. ) ;
#22057=EDGE_CURVE ( 'NONE', #52539, #6658, #35240, .T. ) ;
#22058=CARTESIAN_POINT ( 'NONE',  ( 5.787933236233000045, -76.93448667140100383, -7.442428143219999903 ) ) ;
#22065=VECTOR ( 'NONE', #7014, 1000.000000000000114 ) ;
#22081=DIRECTION ( 'NONE',  ( 0.000000000000000000, -1.000000000000000000, 0.000000000000000000 ) ) ;
#22115=CARTESIAN_POINT ( 'NONE',  ( -8.383077572658999443, -77.65125584965400662, 4.458862939031999595 ) ) ;
#22138=CARTESIAN_POINT ( 'NONE',  ( -9.646812774837000504, -76.86848998579799286, 1.323497712265999882 ) ) ;
#22152=CARTESIAN_POINT ( 'NONE',  ( -5.505695391233000002, -78.64704805011498934, -8.014431902511001127 ) ) ;
#22186=ORIENTED_EDGE ( 'NONE', *, *, #43462, .T. ) ;
#22195=CARTESIAN_POINT ( 'NONE',  ( 9.310971084499998440, -78.40158998579799743, 2.673395725080999874 ) ) ;
#22207=CARTESIAN_POINT ( 'NONE',  ( -9.363446672522654168, -79.41312937742843303, -1.604998447536725603 ) ) ;
#22209=CARTESIAN_POINT ( 'NONE',  ( -2.179156891764956416, -79.40744640124135856, -9.282072619734307750 ) ) ;
#22213=CARTESIAN_POINT ( 'NONE',  ( -6.277317685251144752, -79.23269343647702101, 7.157620870793346413 ) ) ;
#22225=CARTESIAN_POINT ( 'NONE',  ( -2.486604901413152824, -78.40416666666666856, -9.252740428349003565 ) ) ;
#22267=CARTESIAN_POINT ( 'NONE',  ( 0.000000000000000000, -75.20000000000000284, -5.100000000000000533 ) ) ;
#22271=CARTESIAN_POINT ( 'NONE',  ( -1.413089197430621669, -79.28666837594398942, 9.394211990193552353 ) ) ;
#22305=CARTESIAN_POINT ( 'NONE',  ( -2.178743964827522639, -79.00666666666666060, -9.280974303042503593 ) ) ;
#22307=CARTESIAN_POINT ( 'NONE',  ( 5.728183583606999640, -79.68258667140098339, -7.739857582846999762 ) ) ;
#22330=DIRECTION ( 'NONE',  ( 0.000000000000000000, 0.000000000000000000, -1.000000000000000000 ) ) ;
#22342=ORIENTED_EDGE ( 'NONE', *, *, #15656, .F. ) ;
#22347=CARTESIAN_POINT ( 'NONE',  ( 8.250583883964464960, -79.55729166666260710, 4.756314483000303461 ) ) ;
#22358=CARTESIAN_POINT ( 'NONE',  ( 8.737261393354000205, -77.04368667140099092, 4.355473623822999407 ) ) ;
#22365=CARTESIAN_POINT ( 'NONE',  ( 9.539544502573999551, -79.40450095943377562, 0.5400218831817873433 ) ) ;
#22395=CARTESIAN_POINT ( 'NONE',  ( -8.658543215228000633, -79.65891332859899876, 3.968578621617999680 ) ) ;
#22416=CARTESIAN_POINT ( 'NONE',  ( -4.342561293556999935, -77.65714805011499777, -8.443909622126001935 ) ) ;
#22435=CARTESIAN_POINT ( 'NONE',  ( 4.927379535269999167, -77.61086332859899528, -8.272319949952999352 ) ) ;
#22449=CARTESIAN_POINT ( 'NONE',  ( -9.631455446501000495, -78.08089805011499607, -1.333735528292999906 ) ) ;
#22451=CARTESIAN_POINT ( 'NONE',  ( 9.199999999999999289, -76.00000000000000000, 0.000000000000000000 ) ) ;
#22456=CARTESIAN_POINT ( 'NONE',  ( 6.055527902613000002, -78.11999999999999034, 7.319875806370000682 ) ) ;
#22477=ADVANCED_FACE ( 'NONE', ( #19650 ), #2550, .T. ) ;
#22486=CARTESIAN_POINT ( 'NONE',  ( 6.722129540286000626, -77.31653998579800202, -6.773005240843000152 ) ) ;
#22497=CARTESIAN_POINT ( 'NONE',  ( 3.938458446976999205, -79.21000000000000796, -8.369650235310999165 ) ) ;
#22499=VERTEX_POINT ( 'NONE', #50956 ) ;
#22504=DIRECTION ( 'NONE',  ( 0.000000000000000000, 1.000000000000000000, 0.000000000000000000 ) ) ;
#22508=CARTESIAN_POINT ( 'NONE',  ( -6.729900695599003946, -79.46213953550058307, -6.704927793111417955 ) ) ;
#22510=CARTESIAN_POINT ( 'NONE',  ( -3.692575783495599673, -79.39408385515501720, -8.790537166344741138 ) ) ;
#22526=CARTESIAN_POINT ( 'NONE',  ( 1.243547092045970581, -78.43541666666664014, -9.500000000000000000 ) ) ;
#22573=CARTESIAN_POINT ( 'NONE',  ( -9.292587090298047414, -79.38272904684014009, 1.999716160172516632 ) ) ;
#22576=ORIENTED_EDGE ( 'NONE', *, *, #45487, .T. ) ;
#22577=PRODUCT_DEFINITION_FORMATION_WITH_SPECIFIED_SOURCE ( 'ANY', '', #38457, .NOT_KNOWN. ) ;
#22636=B_SPLINE_SURFACE_WITH_KNOTS ( 'NONE', 3, 3, ( 
 ( #3824, #30672, #48708, #7964, #25962, #48995, #8254, #26254, #3259, #25676, #4115, #43985, #21250, #22115, #39252, #31249, #3538, #4413, #53130, #44268, #21540, #49291, #39830, #56980, #39546, #57268, #57842, #40124, #8842, #35692, #57550, #16832, #16542, #34522, #17112 ),
 ( #35096, #52555, #12680, #30093, #10313, #18295, #19167, #36868, #41017, #10022, #50471, #23583, #36290, #31847, #27424, #14718, #892, #9724, #40429, #41598, #28000, #609, #27713, #28292, #46048, #27125, #5573, #1177, #5290, #50767, #18589, #37162, #45165, #31548, #20 ),
 ( #55176, #32715, #13851, #54880, #4715, #22713, #45757, #46343, #40727, #22416, #17999, #45459, #35990, #23297, #49889, #54312, #13556, #41306, #318, #54015, #49595, #9434, #9140, #5002, #23006, #36580, #54602, #14430, #14139, #32138, #50179, #18875, #32425, #34169, #52206 ),
 ( #20051, #6748, #42773, #33602, #51641, #15017, #7039, #56345, #51925, #24173, #11483, #37452, #11196, #51345, #33885, #55469, #10607, #20330, #55770, #20616, #2051, #43061, #47219, #29454, #15316, #46634, #42189, #41890, #38617, #33011, #38039, #25039, #28880, #2619, #6164 ) ),
 .UNSPECIFIED., .F., .F., .F.,
 ( 4, 4 ),
 ( 4, 1, 1, 1, 1, 1, 1, 1, 1, 1, 1, 1, 1, 1, 1, 1, 1, 1, 1, 1, 1, 1, 1, 1, 1, 1, 1, 1, 1, 1, 1, 1, 4 ),
 ( -0.4015584965371999937, 1.401558496537000043 ),
 ( -0.01447761194029999893, 0.009048507462687000596, 0.03257462686566999638, 0.05610074626866000391, 0.07962686567163999862, 0.1031529850746000093, 0.1266791044776000019, 0.1502052238806000084, 0.1737313432835999871, 0.1972574626865999936, 0.2207835820896000001, 0.2443097014925000032, 0.2678358208955000097, 0.2913619402984999884, 0.3148880597015000227, 0.3384141791045000014, 0.3619402985074999801, 0.3854664179103999833, 0.4089925373133999620, 0.4325186567163999962, 0.4560447761193999749, 0.4795708955224000092, 0.5030970149253999324, 0.5266231343284000221, 0.5501492537312999698, 0.5736753731343000595, 0.5972014925372999272, 0.6207276119402999059, 0.6442537313433001067, 0.6677798507462999744, 0.6913059701493000642, 0.7148320895521999008, 0.7383582089551999905 ),
 .UNSPECIFIED. ) ;
#22661=CARTESIAN_POINT ( 'NONE',  ( -8.554185150784999081, -77.36226001420200760, -4.929210599936999948 ) ) ;
#22688=CARTESIAN_POINT ( 'NONE',  ( 9.188870790291838730, -78.07333333333335190, 2.784684813981618490 ) ) ;
#22703=ORIENTED_EDGE ( 'NONE', *, *, #22944, .F. ) ;
#22707=ADVANCED_FACE ( 'NONE', ( #42968 ), #15733, .F. ) ;
#22713=CARTESIAN_POINT ( 'NONE',  ( 8.503129636637000388, -77.78324805011499166, -4.225430575863000193 ) ) ;
#22732=CARTESIAN_POINT ( 'NONE',  ( -7.226567707739000923, -77.32088998579800432, 6.526040278862000221 ) ) ;
#22743=DIRECTION ( 'NONE',  ( -0.7071067811865474617, -0.7071067811865474617, 9.038574250522602634E-10 ) ) ;
#22744=CARTESIAN_POINT ( 'NONE',  ( -9.601739433208001273, -79.02244415034599001, -1.533141744029000053 ) ) ;
#22772=PRESENTATION_STYLE_ASSIGNMENT (( #49949 ) ) ;
#22780=ORIENTED_EDGE ( 'NONE', *, *, #36033, .T. ) ;
#22786=CARTESIAN_POINT ( 'NONE',  ( 4.581254438705999910, -78.79353998579799168, -8.535416510302999527 ) ) ;
#22800=CARTESIAN_POINT ( 'NONE',  ( -7.985521294471968012, -79.44573719447619453, -5.195944220544125081 ) ) ;
#22802=CARTESIAN_POINT ( 'NONE',  ( 0.000000000000000000, -78.00000000000000000, -7.200000000000000178 ) ) ;
#22813=EDGE_CURVE ( 'NONE', #10320, #34146, #18603, .T. ) ;
#22818=CARTESIAN_POINT ( 'NONE',  ( -7.596835002782709623, -78.35208333333333997, -5.838193839761696147 ) ) ;
#22828=CARTESIAN_POINT ( 'NONE',  ( -9.500000000000000000, -77.29999999999999716, 0.000000000000000000 ) ) ;
#22854=VERTEX_POINT ( 'NONE', #42020 ) ;
#22901=CARTESIAN_POINT ( 'NONE',  ( -9.629019889039001967, -79.50708667140099806, -0.02420058354726000241 ) ) ;
#22944=EDGE_CURVE ( 'NONE', #8584, #47685, #15770, .T. ) ;
#22970=DIRECTION ( 'NONE',  ( 0.000000000000000000, 1.000000000000000000, 0.000000000000000000 ) ) ;
#22985=CARTESIAN_POINT ( 'NONE',  ( -4.639000034858584698, -77.00000000000001421, 8.062223707945781470 ) ) ;
#23006=CARTESIAN_POINT ( 'NONE',  ( -1.269916711065999904, -77.18427305011499584, -9.409822520238998678 ) ) ;
#23007=CARTESIAN_POINT ( 'NONE',  ( 0.000000000000000000, -78.00000000000000000, 0.000000000000000000 ) ) ;
#23024=CARTESIAN_POINT ( 'NONE',  ( -1.220391020831000040, -77.26433998579800289, 9.660389656331998864 ) ) ;
#23034=CARTESIAN_POINT ( 'NONE',  ( -0.8481231068849000021, -78.89179415034600140, 9.686304223355000076 ) ) ;
#23089=CARTESIAN_POINT ( 'NONE',  ( 3.324665820279027351, -79.45421531254355330, -8.934852078635632466 ) ) ;
#23114=CARTESIAN_POINT ( 'NONE',  ( 2.411445140827727318, -77.00404005906661098, 8.942079950171093472 ) ) ;
#23121=CARTESIAN_POINT ( 'NONE',  ( 4.846722427696010804, -79.75000000000000000, -7.911989270330391122 ) ) ;
#23175=CARTESIAN_POINT ( 'NONE',  ( 6.644622036202999737, -78.25581001420199811, -7.049129409659999901 ) ) ;
#23212=FACE_OUTER_BOUND ( 'NONE', #56420, .T. ) ;
#23213=VERTEX_POINT ( 'NONE', #12737 ) ;
#23215=EDGE_LOOP ( 'NONE', ( #49805, #10416, #7546, #18497 ) ) ;
#23220=AXIS2_PLACEMENT_3D ( 'NONE', #31268, #4732, #36008 ) ;
#23224=CARTESIAN_POINT ( 'NONE',  ( 9.231185137975039368, -79.16876909680533458, 2.269161111927250563 ) ) ;
#23239=CARTESIAN_POINT ( 'NONE',  ( 7.601898381947000516, -77.37083501420200093, 5.548685371626999263 ) ) ;
#23244=CARTESIAN_POINT ( 'NONE',  ( 9.126301671913999769, -77.41671332859898769, -3.143863093112999607 ) ) ;
#23246=CARTESIAN_POINT ( 'NONE',  ( -1.489189600238929989, -77.01250000000003126, -9.412174122262570108 ) ) ;
#23250=CYLINDRICAL_SURFACE ( 'NONE', #12560, 9.500000000000000000 ) ;
#23274=AXIS2_PLACEMENT_3D ( 'NONE', #16387, #12525, #26096 ) ;
#23277=CARTESIAN_POINT ( 'NONE',  ( -1.923984835444398023, -77.00000000000001421, 9.100276353209897806 ) ) ;
#23280=CARTESIAN_POINT ( 'NONE',  ( 9.448795662942000462, -79.52248667140099769, 1.876396759601000053 ) ) ;
#23297=CARTESIAN_POINT ( 'NONE',  ( -8.383077572658999443, -77.53104805011500389, 4.458862939031999595 ) ) ;
#23309=CARTESIAN_POINT ( 'NONE',  ( -4.784380313523580064, -77.71666666666668277, 8.300970689365431809 ) ) ;
#23313=FACE_OUTER_BOUND ( 'NONE', #17039, .T. ) ;
#23323=ORIENTED_EDGE ( 'NONE', *, *, #35099, .F. ) ;
#23329=CARTESIAN_POINT ( 'NONE',  ( 6.017032375295198854, -77.00000000000000000, 7.093946000275482611 ) ) ;
#23353=CARTESIAN_POINT ( 'NONE',  ( -9.326577543113813817, -76.99999999999998579, -0.5108809166760798215 ) ) ;
#23357=DIRECTION ( 'NONE',  ( 0.000000000000000000, 1.000000000000000000, 0.000000000000000000 ) ) ;
#23363=CARTESIAN_POINT ( 'NONE',  ( -9.193055583834000899, -77.84673998579799559, 3.991918584785999702 ) ) ;
#23407=CARTESIAN_POINT ( 'NONE',  ( -2.712012240502000182, -77.54804903538301630, 9.099584490865000319 ) ) ;
#23431=EDGE_CURVE ( 'NONE', #49808, #25686, #55383, .T. ) ;
#23445=ADVANCED_FACE ( 'NONE', ( #19927 ), #33772, .T. ) ;
#23462=ADVANCED_FACE ( 'NONE', ( #6338 ), #28014, .F. ) ;
#23467=CARTESIAN_POINT ( 'NONE',  ( 0.000000000000000000, -79.79999999999999716, 0.000000000000000000 ) ) ;
#23471=B_SPLINE_CURVE_WITH_KNOTS ( 'NONE', 3,
 ( #48266, #7801, #26085, #25801, #7223, #43828, #38514, #47975, #57672, #12229 ),
 .UNSPECIFIED., .F., .F.,
 ( 4, 2, 2, 2, 4 ),
 ( 0.000000000000000000, 0.2500000000000000000, 0.5000000000000000000, 0.7500000000000000000, 1.000000000000000000 ),
 .UNSPECIFIED. ) ;
#23488=CARTESIAN_POINT ( 'NONE',  ( 1.861092857305999937, -79.77065194988500707, -9.371850619045000386 ) ) ;
#23500=VERTEX_POINT ( 'NONE', #1639 ) ;
#23501=EDGE_CURVE ( 'NONE', #5875, #41593, #14033, .T. ) ;
#23502=LINE ( 'NONE', #29092, #9876 ) ;
#23525=CARTESIAN_POINT ( 'NONE',  ( -7.278018565911000159, -77.62531001420200027, -5.967178069611000168 ) ) ;
#23545=DIRECTION ( 'NONE',  ( 8.742340186909000165E-11, -1.000000000000000000, 2.562965779940999802E-09 ) ) ;
#23564=CARTESIAN_POINT ( 'NONE',  ( -6.709544961267000396, -79.63031332859900147, 6.760325364400999959 ) ) ;
#23583=CARTESIAN_POINT ( 'NONE',  ( -9.061228178001998756, -77.65420194988499247, -2.837532765875999896 ) ) ;
#23585=DIRECTION ( 'NONE',  ( 0.000000000000000000, 0.000000000000000000, -1.000000000000000000 ) ) ;
#23588=CARTESIAN_POINT ( 'NONE',  ( -9.500000000000000000, -78.29999999999999716, 0.000000000000000000 ) ) ;
#23596=VECTOR ( 'NONE', #56324, 1000.000000000000114 ) ;
#23648=CARTESIAN_POINT ( 'NONE',  ( 8.642645349805999189, -78.58708998579800209, -5.074666031188000304 ) ) ;
#23654=CARTESIAN_POINT ( 'NONE',  ( -9.222359558045559069, -79.38018218778096013, 2.295680754222614084 ) ) ;
#23661=AXIS2_PLACEMENT_3D ( 'NONE', #10814, #38238, #37069 ) ;
#23683=DIRECTION ( 'NONE',  ( 0.000000000000000000, 1.000000000000000000, 0.000000000000000000 ) ) ;
#23725=AXIS2_PLACEMENT_3D ( 'NONE', #36740, #45332, #9599 ) ;
#23726=EDGE_CURVE ( 'NONE', #24467, #47685, #26651, .T. ) ;
#23747=CARTESIAN_POINT ( 'NONE',  ( 1.708922835747884506, -77.68932193750340787, -9.291094250111688879 ) ) ;
#23770=CARTESIAN_POINT ( 'NONE',  ( 8.307189301499999345, -79.65391332859900331, -4.458756970628000360 ) ) ;
#23779=CARTESIAN_POINT ( 'NONE',  ( 2.769824414688999870, -79.27925194988499413, -8.825563591736999669 ) ) ;
#23788=CARTESIAN_POINT ( 'NONE',  ( 0.000000000000000000, -75.09999999996229292, -11.54999999996000071 ) ) ;
#23790=VERTEX_POINT ( 'NONE', #21369 ) ;
#23795=ORIENTED_EDGE ( 'NONE', *, *, #887, .T. ) ;
#23814=CARTESIAN_POINT ( 'NONE',  ( 5.196759135519999795, -77.39911001420199455, 7.846684831825000650 ) ) ;
#23819=CARTESIAN_POINT ( 'NONE',  ( 9.361362996599000397, -77.96271332859899417, 2.353468592436000151 ) ) ;
#23864=VERTEX_POINT ( 'NONE', #36984 ) ;
#23891=CARTESIAN_POINT ( 'NONE',  ( -7.160332295859999974, -76.82136498579799877, 6.396111552352999219 ) ) ;
#23923=CARTESIAN_POINT ( 'NONE',  ( 8.718213946067898235, -79.51041666666540664, -3.877033209321456120 ) ) ;
#23927=CARTESIAN_POINT ( 'NONE',  ( -9.240267274125507413, -76.99999999999998579, 1.212345689707036156 ) ) ;
#23937=CARTESIAN_POINT ( 'NONE',  ( 5.365645860858369254, -77.72750000000002046, 7.890595865543486020 ) ) ;
#23957=CARTESIAN_POINT ( 'NONE',  ( -9.400797763902113857, -79.31390857863736699, -1.591501164855807948 ) ) ;
#23960=DIRECTION ( 'NONE',  ( 0.000000000000000000, -1.000000000000000000, 0.000000000000000000 ) ) ;
#23962=AXIS2_PLACEMENT_3D ( 'NONE', #10836, #28812, #6388 ) ;
#23982=B_SPLINE_CURVE_WITH_KNOTS ( 'NONE', 3,
 ( #46007, #1136, #33263, #51304 ),
 .UNSPECIFIED., .F., .F.,
 ( 4, 4 ),
 ( 0.000000000000000000, 1.000000000000000000 ),
 .UNSPECIFIED. ) ;
#24004=CARTESIAN_POINT ( 'NONE',  ( -8.300970689365446020, -77.84166666666669698, -4.784380313523547201 ) ) ;
#24025=CARTESIAN_POINT ( 'NONE',  ( -0.6670706960860000034, -78.20096001420199627, 10.00022801703000042 ) ) ;
#24032=CARTESIAN_POINT ( 'NONE',  ( 9.500000000000000000, -77.64999999999999147, 0.000000000000000000 ) ) ;
#24041=CARTESIAN_POINT ( 'NONE',  ( 8.565463562696219668, -77.26519693750341844, -3.984681137958045571 ) ) ;
#24044=CARTESIAN_POINT ( 'NONE',  ( -3.218338554480999925, -78.16871001420200571, -9.136931980783000284 ) ) ;
#24069=CARTESIAN_POINT ( 'NONE',  ( 0.000000000000000000, -75.10000000019110189, 0.000000000000000000 ) ) ;
#24073=CARTESIAN_POINT ( 'NONE',  ( 5.645287065787000458, -79.39464805011499493, 7.708789581145000014 ) ) ;
#24077=CARTESIAN_POINT ( 'NONE',  ( 7.596835002782696300, -77.20208333333333428, 5.838193839761711246 ) ) ;
#24108=EDGE_CURVE ( 'NONE', #45676, #52926, #43955, .T. ) ;
#24112=CARTESIAN_POINT ( 'NONE',  ( -9.408840690779999960, -77.56876001420199884, 0.2246891580983999825 ) ) ;
#24116=CARTESIAN_POINT ( 'NONE',  ( 8.057735164907999348, -77.48951332859898855, 5.314711785903000418 ) ) ;
#24126=CARTESIAN_POINT ( 'NONE',  ( -7.530775182571000315, -78.12444805011499227, -6.150709233331999037 ) ) ;
#24140=CARTESIAN_POINT ( 'NONE',  ( 1.000000000000000000, -75.20000000000000284, 7.200000000000000178 ) ) ;
#24169=DIRECTION ( 'NONE',  ( 1.000000000000000000, 0.000000000000000000, 0.000000000000000000 ) ) ;
#24173=CARTESIAN_POINT ( 'NONE',  ( -4.342561293556999935, -77.59704415034600800, -8.443909622126001935 ) ) ;
#24174=DIRECTION ( 'NONE',  ( 0.000000000000000000, 1.000000000000000000, 0.000000000000000000 ) ) ;
#24177=CARTESIAN_POINT ( 'NONE',  ( 9.723591721872441695, -78.80042913613843325, 0.1588614647341892172 ) ) ;
#24227=CARTESIAN_POINT ( 'NONE',  ( -5.329221945977861807, -76.99999999999998579, -7.828459959116974787 ) ) ;
#24232=AXIS2_PLACEMENT_3D ( 'NONE', #56395, #15068, #33063 ) ;
#24238=CARTESIAN_POINT ( 'NONE',  ( 4.448768332841000372, -78.71773998579799070, 8.980869306721999124 ) ) ;
#24244=CARTESIAN_POINT ( 'NONE',  ( -9.035542397009781013, -79.37473505568793541, 2.933552591326429315 ) ) ;
#24275=CARTESIAN_POINT ( 'NONE',  ( -3.039602602086000083, -79.28985584965398914, -9.236151215514999180 ) ) ;
#24309=ORIENTED_EDGE ( 'NONE', *, *, #40301, .F. ) ;
#24324=CARTESIAN_POINT ( 'NONE',  ( 10.02101539056000057, -79.07196001420199138, 0.1637206938138999757 ) ) ;
#24338=VECTOR ( 'NONE', #31635, 1000.000000000000000 ) ;
#24346=CARTESIAN_POINT ( 'NONE',  ( -8.838907858698000553, -78.60421001420199616, -3.964206742940000083 ) ) ;
#24365=CARTESIAN_POINT ( 'NONE',  ( 8.400841032887999660, -79.59013998579800386, -4.509023106980999174 ) ) ;
#24370=CARTESIAN_POINT ( 'NONE',  ( -0.5312504855272001114, -78.77064514476064971, -9.708839960653000034 ) ) ;
#24374=CARTESIAN_POINT ( 'NONE',  ( 9.539544502573999551, -79.44465584965399785, 0.5400218831817999998 ) ) ;
#24378=CARTESIAN_POINT ( 'NONE',  ( -1.243547092045993674, -77.28541666666666288, 9.499999999999996447 ) ) ;
#24392=CARTESIAN_POINT ( 'NONE',  ( 6.312739868268272936, -79.21696743740758961, 7.099225441629251065 ) ) ;
#24407=LINE ( 'NONE', #10031, #3329 ) ;
#24420=CARTESIAN_POINT ( 'NONE',  ( 0.000000000000000000, -78.00000000000000000, 0.000000000000000000 ) ) ;
#24457=AXIS2_PLACEMENT_3D ( 'NONE', #52396, #51825, #30221 ) ;
#24467=VERTEX_POINT ( 'NONE', #45183 ) ;
#24527=CARTESIAN_POINT ( 'NONE',  ( 9.633138876124000660, -78.15158998579799743, 2.765897569310999948 ) ) ;
#24530=EDGE_CURVE ( 'NONE', #37512, #233, #26998, .T. ) ;
#24534=CARTESIAN_POINT ( 'NONE',  ( -9.034130664364234065, -79.37469812230315824, 2.937899820749584112 ) ) ;
#24565=CARTESIAN_POINT ( 'NONE',  ( 8.384816012895999648, -78.89790584965399489, -4.923277454554000343 ) ) ;
#24572=ORIENTED_EDGE ( 'NONE', *, *, #45707, .T. ) ;
#24614=CARTESIAN_POINT ( 'NONE',  ( 5.320338141332999982, -79.36539666193300491, -7.841092173349999861 ) ) ;
#24633=CARTESIAN_POINT ( 'NONE',  ( 4.634092916811999530, -78.67108667140098532, -8.633860817301998836 ) ) ;
#24646=( GEOMETRIC_REPRESENTATION_CONTEXT ( 3 ) GLOBAL_UNCERTAINTY_ASSIGNED_CONTEXT ( ( #52006 ) ) GLOBAL_UNIT_ASSIGNED_CONTEXT ( ( #38750, #25751, #16329 ) ) REPRESENTATION_CONTEXT ( 'NONE', 'WORKASPACE' ) );
#24653=CARTESIAN_POINT ( 'NONE',  ( 7.737894983877000143, -79.57843998579799916, -5.744169665113000534 ) ) ;
#24659=CARTESIAN_POINT ( 'NONE',  ( 4.316051676898999823, -78.98839514476064494, 8.712949996777000550 ) ) ;
#24665=CARTESIAN_POINT ( 'NONE',  ( 1.861092857305999937, -79.83075584965399685, -9.371850619045000386 ) ) ;
#24677=VERTEX_POINT ( 'NONE', #51075 ) ;
#24678=ADVANCED_FACE ( 'NONE', ( #42207 ), #55192, .T. ) ;
#24681=CARTESIAN_POINT ( 'NONE',  ( 6.963965595795851726, -79.20918829156502738, 6.469944903610358011 ) ) ;
#24715=CARTESIAN_POINT ( 'NONE',  ( 9.500000000000001776, -78.16041666666667709, 1.243547092045981239 ) ) ;
#24762=CARTESIAN_POINT ( 'NONE',  ( -7.531956854635054377, -78.10362913613842295, -6.151674355925288218 ) ) ;
#24777=ORIENTED_EDGE ( 'NONE', *, *, #7953, .F. ) ;
#24900=CARTESIAN_POINT ( 'NONE',  ( 9.557721383756000222, -78.48558667140099487, -2.621152531184999912 ) ) ;
#24912=CARTESIAN_POINT ( 'NONE',  ( -9.491795480648855587, -79.40409383075655114, -0.5089449881589561686 ) ) ;
#24918=EDGE_CURVE ( 'NONE', #16476, #18472, #9020, .T. ) ;
#24920=CARTESIAN_POINT ( 'NONE',  ( 4.530904210857999992, -77.84363667140100063, 8.688217354640999091 ) ) ;
#24952=CARTESIAN_POINT ( 'NONE',  ( -9.252740428349007118, -77.37916666666666288, 2.486604901413125734 ) ) ;
#24955=CARTESIAN_POINT ( 'NONE',  ( 2.486604901413132840, -78.65416666666668277, 9.252740428349005342 ) ) ;
#24965=CARTESIAN_POINT ( 'NONE',  ( 7.687192023495246218, -79.19968127005114411, 5.581541409190941216 ) ) ;
#24971=CARTESIAN_POINT ( 'NONE',  ( 6.929335342686214538, -79.74160298504301636, -6.198367606484551651 ) ) ;
#24997=CARTESIAN_POINT ( 'NONE',  ( 1.243547092045927949, -78.26458333333332007, 9.500000000000003553 ) ) ;
#25039=CARTESIAN_POINT ( 'NONE',  ( -2.205007487985999770, -76.90349415034600611, 9.235565851336001941 ) ) ;
#25051=CARTESIAN_POINT ( 'NONE',  ( 3.797573017451999711, -78.16306001420198868, 8.745505052098000220 ) ) ;
#25113=( GEOMETRIC_REPRESENTATION_CONTEXT ( 3 ) GLOBAL_UNCERTAINTY_ASSIGNED_CONTEXT ( ( #56717 ) ) GLOBAL_UNIT_ASSIGNED_CONTEXT ( ( #47884, #47601, #7416 ) ) REPRESENTATION_CONTEXT ( 'NONE', 'WORKASPACE' ) );
#25138=CARTESIAN_POINT ( 'NONE',  ( -3.339615680726000235, -78.53295194988498906, 9.131854552393999569 ) ) ;
#25147=CARTESIAN_POINT ( 'NONE',  ( 0.000000000000000000, -75.00000000000000000, 7.200000000000000178 ) ) ;
#25161=AXIS2_PLACEMENT_3D ( 'NONE', #14447, #46066, #50194 ) ;
#25163=VECTOR ( 'NONE', #50141, 1000.000000000000000 ) ;
#25182=CARTESIAN_POINT ( 'NONE',  ( 1.000000000000000000, -78.00000000000000000, -7.200000000000000178 ) ) ;
#25183=CARTESIAN_POINT ( 'NONE',  ( 2.052412689622999942, -78.39848667140098826, -9.695776403646000574 ) ) ;
#25201=CIRCLE ( 'NONE', #16699, 5.100000000000000533 ) ;
#25204=CARTESIAN_POINT ( 'NONE',  ( -0.6521978219530000231, -77.88718667140099683, 9.777264943591001511 ) ) ;
#25209=CARTESIAN_POINT ( 'NONE',  ( 2.486604901413172364, -78.94583333333333997, -9.252740428348998236 ) ) ;
#25252=CIRCLE ( 'NONE', #52557, 11.44999999999999929 ) ;
#25255=CARTESIAN_POINT ( 'NONE',  ( 6.607089402419984658, -79.21351212151715515, 6.827904746749715592 ) ) ;
#25284=LINE ( 'NONE', #43017, #53377 ) ;
#25292=ORIENTED_EDGE ( 'NONE', *, *, #42418, .F. ) ;
#25321=ORIENTED_EDGE ( 'NONE', *, *, #13697, .T. ) ;
#25367=ORIENTED_EDGE ( 'NONE', *, *, #31084, .F. ) ;
#25371=CARTESIAN_POINT ( 'NONE',  ( -1.906106740367999874, -79.86568667140099365, -9.233453574281998755 ) ) ;
#25430=CARTESIAN_POINT ( 'NONE',  ( -9.631455446501000495, -78.20110584965399880, -1.333735528292999906 ) ) ;
#25470=EDGE_CURVE ( 'NONE', #56311, #2750, #39318, .T. ) ;
#25471=CARTESIAN_POINT ( 'NONE',  ( -3.255457669676000254, -78.29116332859899785, -9.242313942619999168 ) ) ;
#25489=CARTESIAN_POINT ( 'NONE',  ( 6.721258625739999992, -78.19203667140099867, -7.130431436203999773 ) ) ;
#25496=CARTESIAN_POINT ( 'NONE',  ( 7.596835002782722057, -78.99791666666668277, -5.838193839761678383 ) ) ;
#25513=CARTESIAN_POINT ( 'NONE',  ( 0.000000000000000000, -79.50000000000000000, -9.499999999999953815 ) ) ;
#25530=CARTESIAN_POINT ( 'NONE',  ( 1.243547092045928615, -78.66458333333332575, 9.500000000000003553 ) ) ;
#25541=CARTESIAN_POINT ( 'NONE',  ( 1.832813866948703074, -79.25953808981230964, 9.323933791568595808 ) ) ;
#25556=CARTESIAN_POINT ( 'NONE',  ( -2.935661446561999899, -79.50000000000000000, -9.035036904803998681 ) ) ;
#25579=ORIENTED_EDGE ( 'NONE', *, *, #58126, .T. ) ;
#25592=CARTESIAN_POINT ( 'NONE',  ( 5.099999999822000696, -75.20000000017779485, -7.534001399281000208E-10 ) ) ;
#25600=CIRCLE ( 'NONE', #198, 9.199999999999999289 ) ;
#25609=CIRCLE ( 'NONE', #53911, 5.299999999999999822 ) ;
#25617=EDGE_CURVE ( 'NONE', #10344, #24467, #3454, .T. ) ;
#25628=CARTESIAN_POINT ( 'NONE',  ( -4.784380313523575623, -78.81666666666669130, 8.300970689365433586 ) ) ;
#25655=CARTESIAN_POINT ( 'NONE',  ( -3.947687142456000053, -79.66548667140099838, 8.787283549286000195 ) ) ;
#25664=B_SPLINE_CURVE_WITH_KNOTS ( 'NONE', 3,
 ( #29390, #24971, #42992, #2833, #38547, #20830, #56852, #34395, #13926, #31921, #36073, #45536, #36362, #54389, #36653, #44943, #45240, #4499, #22497 ),
 .UNSPECIFIED., .F., .F.,
 ( 4, 1, 1, 1, 1, 1, 1, 1, 1, 1, 1, 1, 1, 1, 1, 1, 4 ),
 ( 0.000000000000000000, 0.04500041105014277593, 0.1100003581458013774, 0.1750003052412117677, 0.2400002523368703622, 0.3050001994322810162, 0.3700001465279396107, 0.4350000936233500148, 0.5000000407190086094, 0.5649999878144189580, 0.6299999349100775525, 0.6949998820054882342, 0.7599998291011468288, 0.8249997761965572884, 0.8899997232919678591, 0.9549996703876262316, 1.000000000000000000 ),
 .UNSPECIFIED. ) ;
#25676=CARTESIAN_POINT ( 'NONE',  ( -4.342561293556999935, -77.77735584965398630, -8.443909622126001935 ) ) ;
#25686=VERTEX_POINT ( 'NONE', #16072 ) ;
#25716=CARTESIAN_POINT ( 'NONE',  ( 7.920136950582000068, -77.92325194988499959, 4.778486233528999705 ) ) ;
#25723=VERTEX_POINT ( 'NONE', #16935 ) ;
#25724=AXIS2_PLACEMENT_3D ( 'NONE', #57172, #8163, #7871 ) ;
#25738=FACE_OUTER_BOUND ( 'NONE', #23215, .T. ) ;
#25739=CARTESIAN_POINT ( 'NONE',  ( 5.894914467206975317, -77.93666666666661058, 7.125729969419699827 ) ) ;
#25750=CONICAL_SURFACE ( 'NONE', #56906, 9.349999999968000353, 0.7853981633972997312 ) ;
#25751=( NAMED_UNIT ( * ) PLANE_ANGLE_UNIT ( ) SI_UNIT ( $, .RADIAN. ) );
#25764=CARTESIAN_POINT ( 'NONE',  ( 6.607804308078000233, -79.44368667140099660, -6.725089593472000082 ) ) ;
#25782=CARTESIAN_POINT ( 'NONE',  ( 0.000000000000000000, -75.20000000000000284, 7.200000000000000178 ) ) ;
#25801=CARTESIAN_POINT ( 'NONE',  ( 8.872994237323281297, -79.12000000000000455, -3.510218210012922668 ) ) ;
#25802=VECTOR ( 'NONE', #21854, 1000.000000000000000 ) ;
#25804=EDGE_CURVE ( 'NONE', #25686, #49594, #19513, .T. ) ;
#25812=CARTESIAN_POINT ( 'NONE',  ( 5.684029094576000141, -79.68554415034599003, -7.680196531179999120 ) ) ;
#25830=CARTESIAN_POINT ( 'NONE',  ( -2.145956266024737769, -79.29304659155522472, 9.258292488271512966 ) ) ;
#25847=CARTESIAN_POINT ( 'NONE',  ( -7.992881336352999355, -77.05258667140100215, -5.171618568468999477 ) ) ;
#25858=CARTESIAN_POINT ( 'NONE',  ( 2.486604901413133728, -78.25416666666667709, 9.252740428349007118 ) ) ;
#25899=AXIS2_PLACEMENT_3D ( 'NONE', #124, #23683, #28099 ) ;
#25903=CARTESIAN_POINT ( 'NONE',  ( -1.229229937364078928, -79.61588541666264973, 9.384114583424059575 ) ) ;
#25911=CARTESIAN_POINT ( 'NONE',  ( -9.123604098306000054, -77.28946001420199252, 3.772406241408000405 ) ) ;
#25941=EDGE_LOOP ( 'NONE', ( #8048, #29850, #29586, #28108 ) ) ;
#25944=CARTESIAN_POINT ( 'NONE',  ( -0.6116994581832999600, -79.70066001420198631, 9.722684469059000634 ) ) ;
#25962=CARTESIAN_POINT ( 'NONE',  ( 9.475051992780000987, -77.93498084965399642, -0.6170397550469999270 ) ) ;
#25990=DIRECTION ( 'NONE',  ( 0.000000000000000000, 1.000000000000000000, 0.000000000000000000 ) ) ;
#25995=DIRECTION ( 'NONE',  ( 0.000000000000000000, 1.000000000000000000, 0.000000000000000000 ) ) ;
#25999=CARTESIAN_POINT ( 'NONE',  ( -9.631455446501000495, -78.14100194988499481, -1.333735528292999906 ) ) ;
#26048=CARTESIAN_POINT ( 'NONE',  ( -2.486604901413153268, -77.50416666666664867, -9.252740428348998236 ) ) ;
#26051=CARTESIAN_POINT ( 'NONE',  ( -4.985213779165269976, -79.48073246256258528, -8.086678520982406582 ) ) ;
#26066=CARTESIAN_POINT ( 'NONE',  ( -1.243547092045951041, -78.91458333333333997, -9.500000000000000000 ) ) ;
#26085=CARTESIAN_POINT ( 'NONE',  ( 9.372585790538634498, -79.13499999999999091, -1.790612804732438779 ) ) ;
#26096=DIRECTION ( 'NONE',  ( 0.000000000000000000, 0.000000000000000000, -1.000000000000000000 ) ) ;
#26105=ORIENTED_EDGE ( 'NONE', *, *, #28870, .F. ) ;
#26111=AXIS2_PLACEMENT_3D ( 'NONE', #9666, #16851, #34833 ) ;
#26118=CARTESIAN_POINT ( 'NONE',  ( -0.7691824896752659235, -79.28114364237121947, 9.473166916040263175 ) ) ;
#26127=AXIS2_PLACEMENT_3D ( 'NONE', #41725, #28421, #47055 ) ;
#26143=FACE_OUTER_BOUND ( 'NONE', #55464, .T. ) ;
#26150=DIRECTION ( 'NONE',  ( 1.000000000000000000, 0.000000000000000000, 0.000000000000000000 ) ) ;
#26159=ORIENTED_EDGE ( 'NONE', *, *, #6182, .F. ) ;
#26173=VECTOR ( 'NONE', #19388, 1000.000000000000114 ) ;
#26201=CARTESIAN_POINT ( 'NONE',  ( 4.937899134609000207, -77.58968667140099740, 8.421832810844000150 ) ) ;
#26230=DIRECTION ( 'NONE',  ( 0.000000000000000000, -1.000000000000000000, 0.000000000000000000 ) ) ;
#26244=VECTOR ( 'NONE', #22504, 1000.000000000000000 ) ;
#26254=CARTESIAN_POINT ( 'NONE',  ( 2.962511214703000384, -77.84040584965400456, -9.021140561863999707 ) ) ;
#26291=CARTESIAN_POINT ( 'NONE',  ( 1.899930039692999895, -78.54950584965399685, 9.535935523283001203 ) ) ;
#26316=VECTOR ( 'NONE', #7505, 1000.000000000000000 ) ;
#26344=CARTESIAN_POINT ( 'NONE',  ( -7.594691572176750505, -79.24835172787872750, 5.837024335811811682 ) ) ;
#26352=DIRECTION ( 'NONE',  ( 1.000000000000000000, 0.000000000000000000, 0.000000000000000000 ) ) ;
#26370=VECTOR ( 'NONE', #37444, 1000.000000000000000 ) ;
#26395=CARTESIAN_POINT ( 'NONE',  ( 0.000000000000000000, -79.65000000003199432, -9.349999999968000353 ) ) ;
#26400=CARTESIAN_POINT ( 'NONE',  ( -5.582146761189269668, -79.32488193069980298, 7.686897053185122175 ) ) ;
#26423=DIRECTION ( 'NONE',  ( 0.000000000000000000, 0.000000000000000000, -1.000000000000000000 ) ) ;
#26431=CARTESIAN_POINT ( 'NONE',  ( 0.1977897354609805813, -79.02666666666665662, -9.531227019568570213 ) ) ;
#26479=CONICAL_SURFACE ( 'NONE', #1091, 5.599999999950999729, 0.2449786631268792425 ) ;
#26480=CARTESIAN_POINT ( 'NONE',  ( 8.780483330769000005, -76.97088667140099005, -4.267527838117000094 ) ) ;
#26554=CARTESIAN_POINT ( 'NONE',  ( -8.488083377859000578, -76.90398832859899869, 4.545599397691000298 ) ) ;
#26564=CARTESIAN_POINT ( 'NONE',  ( 6.218034014419081323, -77.00000000000001421, 6.922517326502717339 ) ) ;
#26567=CARTESIAN_POINT ( 'NONE',  ( -7.603664017118000551, -78.45629415034599674, 6.060370778711000384 ) ) ;
#26617=CARTESIAN_POINT ( 'NONE',  ( -9.500000000000000000, -78.39999999999999147, 0.000000000000000000 ) ) ;
#26621=CARTESIAN_POINT ( 'NONE',  ( -8.709378738715637169, -79.43268344339898590, -3.800117602320954635 ) ) ;
#26639=CARTESIAN_POINT ( 'NONE',  ( 5.838193839761705917, -78.47708333333333997, -7.596835002782701629 ) ) ;
#26641=DIRECTION ( 'NONE',  ( -0.7071067811865474617, -0.7071067811865474617, 1.396797134838093180E-09 ) ) ;
#26651=LINE ( 'NONE', #21658, #39323 ) ;
#26690=CARTESIAN_POINT ( 'NONE',  ( -2.442127856336522296, -79.29558379175310279, 9.187477159757261091 ) ) ;
#26706=CARTESIAN_POINT ( 'NONE',  ( 9.442000951725852076, -77.80242193750341073, 0.3056363532403006955 ) ) ;
#26725=CARTESIAN_POINT ( 'NONE',  ( -3.692578928296568641, -78.99333333333336782, -8.789099506565383635 ) ) ;
#26728=CARTESIAN_POINT ( 'NONE',  ( 8.461214143919999486, -79.29648667140099860, 4.596358662803000428 ) ) ;
#26731=CARTESIAN_POINT ( 'NONE',  ( 3.938458446976999205, -79.21000000000000796, -8.369650235310999165 ) ) ;
#26775=CARTESIAN_POINT ( 'NONE',  ( 5.853183942465999934, -76.99826001420200328, -7.526330923816999530 ) ) ;
#26809=ORIENTED_EDGE ( 'NONE', *, *, #31115, .F. ) ;
#26844=CARTESIAN_POINT ( 'NONE',  ( 2.486604901413132840, -77.65416666666668277, 9.252740428349005342 ) ) ;
#26850=CARTESIAN_POINT ( 'NONE',  ( 7.685661446562000343, -77.00000000000000000, -5.583959896779000509 ) ) ;
#26854=CARTESIAN_POINT ( 'NONE',  ( 9.130836692535000410, -77.66741332859899671, -3.055844195858999690 ) ) ;
#26868=CARTESIAN_POINT ( 'NONE',  ( 9.345760913908002010, -78.34219805011500171, 2.683384691900000174 ) ) ;
#26903=CARTESIAN_POINT ( 'NONE',  ( -9.193191990781000911, -77.60773998579799127, 2.558485205664000173 ) ) ;
#26909=CARTESIAN_POINT ( 'NONE',  ( -8.988089064694998243, -78.16051332859899503, 3.902915570549000179 ) ) ;
#26910=DIRECTION ( 'NONE',  ( 0.000000000000000000, -1.000000000000000000, 0.000000000000000000 ) ) ;
#26917=CARTESIAN_POINT ( 'NONE',  ( 5.838193839761703252, -77.57708333333330586, -7.596835002782702517 ) ) ;
#26921=CARTESIAN_POINT ( 'NONE',  ( -6.690353498881652428, -79.46262472211189731, -6.744430746908721908 ) ) ;
#26922=DIRECTION ( 'NONE',  ( 0.000000000000000000, -1.000000000000000000, 0.000000000000000000 ) ) ;
#26945=CARTESIAN_POINT ( 'NONE',  ( -8.123853732960998997, -77.10669903538303060, 4.915330883505999893 ) ) ;
#26948=CARTESIAN_POINT ( 'NONE',  ( -2.486604901413152824, -77.40416666666668277, -9.252740428349003565 ) ) ;
#26969=DIRECTION ( 'NONE',  ( 0.000000000000000000, 0.000000000000000000, -1.000000000000000000 ) ) ;
#26978=ORIENTED_EDGE ( 'NONE', *, *, #36033, .F. ) ;
#26985=CARTESIAN_POINT ( 'NONE',  ( -7.966670494143397008, -79.35374996792596392, 5.181185574044002706 ) ) ;
#26997=AXIS2_PLACEMENT_3D ( 'NONE', #7571, #20575, #30278 ) ;
#26998=CIRCLE ( 'NONE', #23220, 1.000000000000000000 ) ;
#27012=CARTESIAN_POINT ( 'NONE',  ( 0.000000000000000000, -75.10000000019110189, 0.000000000000000000 ) ) ;
#27028=CARTESIAN_POINT ( 'NONE',  ( 3.938458446976999205, -79.30999999999998806, -8.369650235310999165 ) ) ;
#27040=B_SPLINE_CURVE_WITH_KNOTS ( 'NONE', 3,
 ( #40073, #4061, #4668, #35940, #53968, #12913, #57795, #4365, #53666, #58089, #31200, #22365, #17351, #44225, #13206, #31497 ),
 .UNSPECIFIED., .F., .F.,
 ( 4, 1, 1, 1, 1, 1, 1, 1, 1, 1, 1, 1, 1, 4 ),
 ( 0.000000000000000000, 0.06727065942882816396, 0.1470435203315429151, 0.2268163812345619923, 0.3065892421372763965, 0.3863621030402955014, 0.4661349639430099057, 0.5459078248460289551, 0.6256806857487438034, 0.7054535466517628528, 0.7852264075544772570, 0.8649992684571919943, 0.9447721293602107107, 1.000000000000000000 ),
 .UNSPECIFIED. ) ;
#27069=CARTESIAN_POINT ( 'NONE',  ( 8.879470778449000790, -77.03466001420198950, -4.315638138276999491 ) ) ;
#27125=CARTESIAN_POINT ( 'NONE',  ( -4.802567994450000377, -77.21285194988500677, -8.191018798270000900 ) ) ;
#27136=CARTESIAN_POINT ( 'NONE',  ( 9.500000000000000000, -77.54999999999999716, 0.000000000000000000 ) ) ;
#27143=CARTESIAN_POINT ( 'NONE',  ( 9.370759595542999421, -77.15123998579800002, 2.646005887749999896 ) ) ;
#27153=CARTESIAN_POINT ( 'NONE',  ( 5.778006553106726173, -77.00000000000000000, 7.287267006099804156 ) ) ;
#27156=CARTESIAN_POINT ( 'NONE',  ( 9.377128579935000374, -78.23854415034598730, -2.571625947824999869 ) ) ;
#27188=CARTESIAN_POINT ( 'NONE',  ( -9.252740428349001789, -78.42083333333334849, -2.486604901413163926 ) ) ;
#27189=CARTESIAN_POINT ( 'NONE',  ( 8.681495883089000998, -76.90711332859899585, -4.219417537955999720 ) ) ;
#27199=CARTESIAN_POINT ( 'NONE',  ( -3.327183877592000183, -78.53223998579800025, 9.097860994781999722 ) ) ;
#27212=CARTESIAN_POINT ( 'NONE',  ( -9.376751323929733317, -79.41245819630034930, -1.524018823012485813 ) ) ;
#27237=CARTESIAN_POINT ( 'NONE',  ( -7.591316436381998933, -77.20127403538302246, -5.703451837412999659 ) ) ;
#27285=CARTESIAN_POINT ( 'NONE',  ( -2.858407197967999913, -79.75000000000000000, -8.797272775729998884 ) ) ;
#27320=CARTESIAN_POINT ( 'NONE',  ( -6.100417943526999842, -79.57728667140099788, -7.450071050714999643 ) ) ;
#27364=VECTOR ( 'NONE', #52026, 1000.000000000000000 ) ;
#27366=DIRECTION ( 'NONE',  ( 1.044282280788000023E-09, -1.000000000000000000, -6.141137129051000072E-09 ) ) ;
#27401=CARTESIAN_POINT ( 'NONE',  ( -5.818047344251811026, -77.00000000000000000, 7.195567332808626482 ) ) ;
#27416=EDGE_CURVE ( 'NONE', #23213, #3012, #2494, .T. ) ;
#27422=AXIS2_PLACEMENT_3D ( 'NONE', #42415, #1686, #28810 ) ;
#27424=CARTESIAN_POINT ( 'NONE',  ( -6.013262726775999489, -77.55962694988500061, 7.348341287529000176 ) ) ;
#27433=CARTESIAN_POINT ( 'NONE',  ( 9.499999999999998224, -77.56041666666668277, 1.243547092045980129 ) ) ;
#27441=CARTESIAN_POINT ( 'NONE',  ( -5.759424782279999988, -77.01708832859898735, -7.716175674550000529 ) ) ;
#27449=CARTESIAN_POINT ( 'NONE',  ( 9.438215368887679091, -77.00000000000000000, -0.5776839348911854133 ) ) ;
#27451=CARTESIAN_POINT ( 'NONE',  ( -0.5312504855272001114, -78.69059805011499975, -9.708839960653000034 ) ) ;
#27485=CARTESIAN_POINT ( 'NONE',  ( -2.489097927752999873, -77.02533998579799857, 9.212221160641000495 ) ) ;
#27529=CARTESIAN_POINT ( 'NONE',  ( -0.7479529023059999782, -77.76872403538301626, -9.465622776916999825 ) ) ;
#27558=ORIENTED_EDGE ( 'NONE', *, *, #30419, .T. ) ;
#27575=CARTESIAN_POINT ( 'NONE',  ( 0.000000000000000000, -75.10000000284179578, 7.200000000000000178 ) ) ;
#27584=CARTESIAN_POINT ( 'NONE',  ( -9.359285000798275078, -77.03899693750341271, 1.284050242927868624 ) ) ;
#27589=CARTESIAN_POINT ( 'NONE',  ( 9.310971084499998440, -78.34291001420200473, 2.673395725080999874 ) ) ;
#27607=CARTESIAN_POINT ( 'NONE',  ( 1.828070329658999960, -79.36668667140099842, 9.453928736856999748 ) ) ;
#27633=ORIENTED_EDGE ( 'NONE', *, *, #18739, .T. ) ;
#27653=CARTESIAN_POINT ( 'NONE',  ( 3.878365675696000103, -77.22946001420200446, -8.575257901267999472 ) ) ;
#27658=CARTESIAN_POINT ( 'NONE',  ( 7.574740816159999390, -77.88991332859899330, -5.983027492110999823 ) ) ;
#27693=CARTESIAN_POINT ( 'NONE',  ( -0.5912419659665999472, -79.50933998579799322, 9.397521941627999809 ) ) ;
#27713=CARTESIAN_POINT ( 'NONE',  ( 5.807838419657000095, -77.30742694988499863, -7.511754867730999763 ) ) ;
#27731=CARTESIAN_POINT ( 'NONE',  ( 0.6755009196905999991, -77.00986498579798933, -9.713710972472000549 ) ) ;
#27747=DIRECTION ( 'NONE',  ( -0.2425356250363094601, 0.9701425001453377606, -4.828653421726189663E-10 ) ) ;
#27768=CARTESIAN_POINT ( 'NONE',  ( -9.218146263507760452, -77.00000000000000000, -1.688195841058859559 ) ) ;
#27775=ORIENTED_EDGE ( 'NONE', *, *, #47199, .T. ) ;
#27776=CARTESIAN_POINT ( 'NONE',  ( -3.133069020688000084, -78.97903998579799634, -9.520158728599000142 ) ) ;
#27793=EDGE_CURVE ( 'NONE', #15664, #21408, #38807, .T. ) ;
#27798=FACE_BOUND ( 'NONE', #44131, .T. ) ;
#27819=CARTESIAN_POINT ( 'NONE',  ( -1.269916711065999904, -77.26432403538302651, -9.409822520238998678 ) ) ;
#27832=EDGE_CURVE ( 'NONE', #29780, #42095, #11023, .T. ) ;
#27863=EDGE_CURVE ( 'NONE', #56311, #34611, #47913, .T. ) ;
#27877=CARTESIAN_POINT ( 'NONE',  ( 9.797588846018999931, -78.75818667140099194, 0.1600704101387999956 ) ) ;
#27894=CARTESIAN_POINT ( 'NONE',  ( 1.918320629100999763, -79.51993998579798983, -9.660030828008999038 ) ) ;
#27905=CARTESIAN_POINT ( 'NONE',  ( 8.150225256662000817, -79.78074805011499393, -4.374508917085999649 ) ) ;
#27922=AXIS2_PLACEMENT_3D ( 'NONE', #5332, #359, #31594 ) ;
#27941=CARTESIAN_POINT ( 'NONE',  ( 8.813612208106999191, -77.78773667140100656, 3.598911935278999774 ) ) ;
#27949=CARTESIAN_POINT ( 'NONE',  ( 0.7491852396053489960, -77.03125000000001421, -9.499759410111733970 ) ) ;
#27982=CARTESIAN_POINT ( 'NONE',  ( 6.121779332999000900, -79.43668667140099160, -7.438015166080000462 ) ) ;
#27984=EDGE_LOOP ( 'NONE', ( #44638, #54990, #46773, #25579 ) ) ;
#28000=CARTESIAN_POINT ( 'NONE',  ( 9.426477049435000310, -77.37047694988500268, -1.139727483088999849 ) ) ;
#28014=CONICAL_SURFACE ( 'NONE', #11070, 1.099999997158000120, 0.7853981633972997312 ) ;
#28032=CARTESIAN_POINT ( 'NONE',  ( -5.099999999822000696, -75.20000000017779485, 7.533999751109999828E-10 ) ) ;
#28049=AXIS2_PLACEMENT_3D ( 'NONE', #38833, #33812, #29100 ) ;
#28059=VECTOR ( 'NONE', #58203, 1000.000000000000114 ) ;
#28066=CARTESIAN_POINT ( 'NONE',  ( -9.943323471430000282, -78.36933998579799265, 1.256133873833999992 ) ) ;
#28071=CARTESIAN_POINT ( 'NONE',  ( -9.048147692728329972, -79.37506682946143144, 2.894494549572617093 ) ) ;
#28077=ORIENTED_EDGE ( 'NONE', *, *, #40025, .T. ) ;
#28092=CARTESIAN_POINT ( 'NONE',  ( 4.784911713602124195, -79.13352425759953235, 8.302150867234010079 ) ) ;
#28099=DIRECTION ( 'NONE',  ( 1.000000000000000000, 0.000000000000000000, 0.000000000000000000 ) ) ;
#28108=ORIENTED_EDGE ( 'NONE', *, *, #31993, .T. ) ;
#28119=CARTESIAN_POINT ( 'NONE',  ( 0.000000000000000000, -74.70999999999999375, 0.000000000000000000 ) ) ;
#28145=CARTESIAN_POINT ( 'NONE',  ( 8.642645349805999189, -79.02841001420199518, -5.074666031188000304 ) ) ;
#28162=CARTESIAN_POINT ( 'NONE',  ( 3.892964293701162592, -77.20864693750340280, -8.607536166100398844 ) ) ;
#28167=CARTESIAN_POINT ( 'NONE',  ( -7.374059913654000376, -79.12681001420199323, -6.282030610069000431 ) ) ;
#28174=DIRECTION ( 'NONE',  ( 1.000000000000000000, 0.000000000000000000, 0.000000000000000000 ) ) ;
#28191=CARTESIAN_POINT ( 'NONE',  ( 4.067416459488999436, -79.29095194988499884, -8.418325902196000854 ) ) ;
#28195=DIRECTION ( 'NONE',  ( -1.000000000000000000, 0.000000000000000000, 0.000000000000000000 ) ) ;
#28196=CARTESIAN_POINT ( 'NONE',  ( -9.500000000000000000, -77.39999999999999147, 0.000000000000000000 ) ) ;
#28202=CARTESIAN_POINT ( 'NONE',  ( 9.500000000000000000, -78.04999999999999716, 0.000000000000000000 ) ) ;
#28219=CARTESIAN_POINT ( 'NONE',  ( 0.000000000000000000, -75.00000000000000000, 6.000000000000230038 ) ) ;
#28221=VECTOR ( 'NONE', #9581, 1000.000000000000000 ) ;
#28225=DIRECTION ( 'NONE',  ( 0.000000000000000000, -1.000000000000000000, 0.000000000000000000 ) ) ;
#28231=CARTESIAN_POINT ( 'NONE',  ( 9.406593443539000177, -77.82323501420199818, 0.3044902167661999726 ) ) ;
#28266=ORIENTED_EDGE ( 'NONE', *, *, #25804, .F. ) ;
#28280=DIRECTION ( 'NONE',  ( 0.000000000000000000, 0.000000000000000000, -1.000000000000000000 ) ) ;
#28292=CARTESIAN_POINT ( 'NONE',  ( 2.459440699436000077, -77.27590194988499661, -9.171074077620000153 ) ) ;
#28347=CARTESIAN_POINT ( 'NONE',  ( -9.331242083993144476, -76.99999999999998579, -0.3638479554798288440 ) ) ;
#28358=CARTESIAN_POINT ( 'NONE',  ( -5.773189589619000195, -77.80318998579799938, 8.192511063987998554 ) ) ;
#28362=CARTESIAN_POINT ( 'NONE',  ( -7.678698829008310689, -79.34948846491148799, 5.593101447762748535 ) ) ;
#28387=VECTOR ( 'NONE', #8126, 1000.000000000000114 ) ;
#28421=DIRECTION ( 'NONE',  ( 0.000000000000000000, 1.000000000000000000, 0.000000000000000000 ) ) ;
#28451=EDGE_CURVE ( 'NONE', #31238, #42268, #43986, .T. ) ;
#28458=CARTESIAN_POINT ( 'NONE',  ( -7.011176471748147954, -77.49139693750339575, 6.331528591067105971 ) ) ;
#28459=COLOUR_RGB ( '', 0.31764706, 0.68627451, 0.89019608) ;
#28462=CARTESIAN_POINT ( 'NONE',  ( 9.685875573750999834, -78.82196001420199138, 0.1582452683012000039 ) ) ;
#28490=CARTESIAN_POINT ( 'NONE',  ( 1.813979036992999783, -79.42974805011499484, 9.381055131006998948 ) ) ;
#28528=CARTESIAN_POINT ( 'NONE',  ( 0.6529096706351000812, -77.20118501420199664, -9.388848551955000232 ) ) ;
#28533=CARTESIAN_POINT ( 'NONE',  ( 4.882231352572000027, -77.52591332859900319, 8.326888637120999803 ) ) ;
#28546=CARTESIAN_POINT ( 'NONE',  ( 5.279327442448000340, -79.18212748368000575, -7.780650776298999816 ) ) ;
#28561=CIRCLE ( 'NONE', #33279, 1.000000000000000000 ) ;
#28582=CIRCLE ( 'NONE', #25724, 5.100000000000000533 ) ;
#28590=DIRECTION ( 'NONE',  ( -1.000000000000000000, 0.000000000000000000, 0.000000000000000000 ) ) ;
#28600=CARTESIAN_POINT ( 'NONE',  ( 9.500000000000001776, -78.13958333333333428, -1.243547092045940827 ) ) ;
#28653=CARTESIAN_POINT ( 'NONE',  ( 2.951189771924322081, -77.75000000000000000, 9.074256859245707574 ) ) ;
#28706=B_SPLINE_CURVE_WITH_KNOTS ( 'NONE', 3,
 ( #46104, #32480, #37213, #28936, #54653, #24227, #55226, #14772, #32771, #50818, #1811, #46396, #36922, #19806, #5060, #9779, #37800, #10361, #5344, #55821, #27768, #54934, #45810, #23353, #18930, #50523, #28347, #5922, #19509, #23927, #41946, #1517, #20382, #34510, #33653, #11815, #42822, #52541, #51693, #21239, #34224, #52258, #38956 ),
 .UNSPECIFIED., .F., .F.,
 ( 4, 2, 2, 2, 2, 1, 2, 2, 1, 2, 2, 1, 1, 1, 1, 2, 2, 1, 1, 1, 1, 2, 2, 1, 2, 2, 4 ),
 ( 0.000000000000000000, 0.06250000000000005551, 0.1250000000000001110, 0.1875000000000001665, 0.2500000000000002220, 0.3125000000000002776, 0.3437500000000001665, 0.3750000000000001110, 0.4375000000000001110, 0.4687500000000001665, 0.5000000000000002220, 0.5625000000000002220, 0.5937500000000003331, 0.6093750000000003331, 0.6171875000000003331, 0.6210937500000003331, 0.6250000000000003331, 0.6875000000000003331, 0.7187500000000004441, 0.7343750000000004441, 0.7421875000000004441, 0.7460937500000004441, 0.7500000000000004441, 0.8125000000000003331, 0.8437500000000003331, 0.8750000000000002220, 1.000000000000000000 ),
 .UNSPECIFIED. ) ;
#28707=ORIENTED_EDGE ( 'NONE', *, *, #11589, .T. ) ;
#28750=CARTESIAN_POINT ( 'NONE',  ( -7.305413871501877487, -77.60449693750338440, -5.989639219614036669 ) ) ;
#28754=CARTESIAN_POINT ( 'NONE',  ( 6.533310722863999942, -79.19368667140099660, -6.649273783659000792 ) ) ;
#28776=CARTESIAN_POINT ( 'NONE',  ( -6.207771380439999653, -79.37311332859900403, 7.503906557766999441 ) ) ;
#28781=CARTESIAN_POINT ( 'NONE',  ( 8.219513559211000242, -78.94484514476064874, 5.194554602171000290 ) ) ;
#28785=CARTESIAN_POINT ( 'NONE',  ( -2.364557222828000072, -79.58505584965399748, 9.257622954664000758 ) ) ;
#28789=CARTESIAN_POINT ( 'NONE',  ( 1.478685787649352434, -79.59375000137556810, -9.318529369750295999 ) ) ;
#28790=ORIENTED_EDGE ( 'NONE', *, *, #58126, .F. ) ;
#28802=CARTESIAN_POINT ( 'NONE',  ( 7.704680120202406890, -79.19943945225395510, 5.557390998954779171 ) ) ;
#28810=DIRECTION ( 'NONE',  ( 0.000000000000000000, 0.000000000000000000, -1.000000000000000000 ) ) ;
#28812=DIRECTION ( 'NONE',  ( 0.000000000000000000, 1.000000000000000000, 0.000000000000000000 ) ) ;
#28870=EDGE_CURVE ( 'NONE', #56311, #2750, #18590, .T. ) ;
#28880=CARTESIAN_POINT ( 'NONE',  ( 1.529609450199000076, -76.87196915034600408, 9.371081266747001592 ) ) ;
#28884=B_SPLINE_CURVE_WITH_KNOTS ( 'NONE', 3,
 ( #14957, #6982, #56291, #51870, #51585, #56003, #47163, #1998, #20564, #33250, #16138, #41836, #2563, #34113, #19401, #11714, #42715, #29691 ),
 .UNSPECIFIED., .F., .F.,
 ( 4, 2, 2, 2, 2, 2, 2, 2, 4 ),
 ( 0.000000000000000000, 0.1250000000000000278, 0.2500000000000000555, 0.3750000000000001110, 0.5000000000000001110, 0.6250000000000001110, 0.7500000000000002220, 0.8750000000000001110, 1.000000000000000000 ),
 .UNSPECIFIED. ) ;
#28888=APPLICATION_CONTEXT ( 'automotive_design' ) ;
#28898=CARTESIAN_POINT ( 'NONE',  ( -1.243547092045993674, -78.78541666666666288, 9.499999999999996447 ) ) ;
#28936=CARTESIAN_POINT ( 'NONE',  ( -4.345263384820875707, -76.99999999999998579, -8.432632365033661870 ) ) ;
#28947=CARTESIAN_POINT ( 'NONE',  ( 6.786979366286999493, -78.19513998579799363, 7.374582364394999701 ) ) ;
#28952=CARTESIAN_POINT ( 'NONE',  ( -9.500094076791862463, -79.39994338716823563, -4.328536937075411965E-07 ) ) ;
#28973=DIRECTION ( 'NONE',  ( 0.7071067811864976127, -0.7071067811865975328, -2.089956507868993372E-09 ) ) ;
#28974=EDGE_CURVE ( 'NONE', #23500, #52926, #53510, .T. ) ;
#28976=ORIENTED_EDGE ( 'NONE', *, *, #35611, .F. ) ;
#29006=ORIENTED_EDGE ( 'NONE', *, *, #13370, .T. ) ;
#29018=EDGE_CURVE ( 'NONE', #22005, #6658, #31343, .T. ) ;
#29029=ORIENTED_EDGE ( 'NONE', *, *, #43247, .T. ) ;
#29035=CARTESIAN_POINT ( 'NONE',  ( 8.472259919707001430, -79.11551001420200180, 5.354284829591000161 ) ) ;
#29048=CARTESIAN_POINT ( 'NONE',  ( -0.9686576707075671422, -79.75000000000000000, -9.250000010076565360 ) ) ;
#29052=CARTESIAN_POINT ( 'NONE',  ( 7.103190263045000563, -77.81460333806700191, 6.271635551916999951 ) ) ;
#29071=CARTESIAN_POINT ( 'NONE',  ( -8.817171295982999979, -79.40821332859900394, 4.135520484479999759 ) ) ;
#29076=CARTESIAN_POINT ( 'NONE',  ( 3.441164836547143668, -77.99567685992036559, 8.842878308218095285 ) ) ;
#29080=CARTESIAN_POINT ( 'NONE',  ( -6.090475762158000350, -79.56005194988499341, 7.362120511650999788 ) ) ;
#29084=CARTESIAN_POINT ( 'NONE',  ( 7.483407197968000801, -79.75000000000000000, -5.437013583705000208 ) ) ;
#29091=EDGE_LOOP ( 'NONE', ( #41315, #3126, #18096, #48495, #10, #21409 ) ) ;
#29092=CARTESIAN_POINT ( 'NONE',  ( -11.65000000000000036, -76.00000000000000000, 0.000000000000000000 ) ) ;
#29095=EDGE_LOOP ( 'NONE', ( #11976, #36210, #34890, #28266 ) ) ;
#29097=CARTESIAN_POINT ( 'NONE',  ( 6.164680649823143455, -79.21867059585197524, 7.228082388273737280 ) ) ;
#29100=DIRECTION ( 'NONE',  ( 0.000000000000000000, 0.000000000000000000, -1.000000000000000000 ) ) ;
#29101=ORIENTED_EDGE ( 'NONE', *, *, #22944, .T. ) ;
#29164=CARTESIAN_POINT ( 'NONE',  ( 1.835192269501999984, -76.98893998579799813, 9.364437132986999757 ) ) ;
#29172=CYLINDRICAL_SURFACE ( 'NONE', #10503, 9.500000000000000000 ) ;
#29182=EDGE_CURVE ( 'NONE', #52771, #1911, #39314, .T. ) ;
#29204=ORIENTED_EDGE ( 'NONE', *, *, #49913, .F. ) ;
#29217=EDGE_CURVE ( 'NONE', #25686, #233, #54254, .T. ) ;
#29228=ORIENTED_EDGE ( 'NONE', *, *, #12558, .F. ) ;
#29233=ORIENTED_EDGE ( 'NONE', *, *, #34661, .F. ) ;
#29279=DIRECTION ( 'NONE',  ( 0.000000000000000000, 1.000000000000000000, 0.000000000000000000 ) ) ;
#29289=AXIS2_PLACEMENT_3D ( 'NONE', #17427, #25990, #12988 ) ;
#29303=ORIENTED_EDGE ( 'NONE', *, *, #12027, .T. ) ;
#29308=ORIENTED_EDGE ( 'NONE', *, *, #14549, .T. ) ;
#29314=CARTESIAN_POINT ( 'NONE',  ( 4.399173910654000430, -79.09528667140098435, 8.880751478442000746 ) ) ;
#29334=CARTESIAN_POINT ( 'NONE',  ( -9.832476300866000329, -78.43311332859899210, 1.242130619674999936 ) ) ;
#29340=CARTESIAN_POINT ( 'NONE',  ( -2.486604901413152824, -78.90416666666666856, -9.252740428349003565 ) ) ;
#29343=CARTESIAN_POINT ( 'NONE',  ( 0.000000000000000000, -74.70999999999999375, 0.000000000000000000 ) ) ;
#29365=CARTESIAN_POINT ( 'NONE',  ( 6.479078291783999966, -79.19414415034599131, -7.022474634662000170 ) ) ;
#29383=CARTESIAN_POINT ( 'NONE',  ( 6.261610633530541037, -79.21755913019184447, 7.144501166461902919 ) ) ;
#29390=CARTESIAN_POINT ( 'NONE',  ( 7.483407197968000801, -79.75000000000000000, -5.437013583705000208 ) ) ;
#29454=CARTESIAN_POINT ( 'NONE',  ( 2.459440699436000077, -77.15569415034599388, -9.171074077620000153 ) ) ;
#29457=ADVANCED_FACE ( 'NONE', ( #6694 ), #15843, .T. ) ;
#29467=FACE_OUTER_BOUND ( 'NONE', #41807, .T. ) ;
#29492=AXIS2_PLACEMENT_3D ( 'NONE', #52288, #11847, #30690 ) ;
#29503=AXIS2_PLACEMENT_3D ( 'NONE', #52603, #3014, #8585 ) ;
#29528=CARTESIAN_POINT ( 'NONE',  ( 0.000000000000000000, -79.50000000000000000, 0.000000000000000000 ) ) ;
#29539=AXIS2_PLACEMENT_3D ( 'NONE', #33711, #29279, #51167 ) ;
#29558=CARTESIAN_POINT ( 'NONE',  ( 7.920136950582000068, -77.98335584965398937, 4.778486233528999705 ) ) ;
#29586=ORIENTED_EDGE ( 'NONE', *, *, #19172, .F. ) ;
#29601=CARTESIAN_POINT ( 'NONE',  ( 6.635658238781000584, -78.50891332859899308, 7.210160158573999389 ) ) ;
#29605=ORIENTED_EDGE ( 'NONE', *, *, #27793, .T. ) ;
#29622=CARTESIAN_POINT ( 'NONE',  ( -9.816946295765999864, -77.95406332859900544, -1.359421753724999959 ) ) ;
#29651=CARTESIAN_POINT ( 'NONE',  ( 8.857115352654000517, -79.22924415034600543, -3.584237475251999872 ) ) ;
#29665=ADVANCED_FACE ( 'NONE', ( #50642 ), #46071, .F. ) ;
#29669=CARTESIAN_POINT ( 'NONE',  ( 4.302121030171025318, -79.23722901812243435, 8.469798634234269485 ) ) ;
#29687=EDGE_CURVE ( 'NONE', #36499, #10154, #43221, .T. ) ;
#29691=CARTESIAN_POINT ( 'NONE',  ( -9.500000000000000000, -77.29999999999999716, 0.000000000000000000 ) ) ;
#29700=FACE_OUTER_BOUND ( 'NONE', #17919, .T. ) ;
#29737=ORIENTED_EDGE ( 'NONE', *, *, #16724, .F. ) ;
#29742=DIRECTION ( 'NONE',  ( 1.000000000000000000, 0.000000000000000000, 0.000000000000000000 ) ) ;
#29749=CARTESIAN_POINT ( 'NONE',  ( 9.252740428349001789, -78.12916666666666288, -2.486604901413144830 ) ) ;
#29780=VERTEX_POINT ( 'NONE', #10601 ) ;
#29783=CARTESIAN_POINT ( 'NONE',  ( -8.855994692495000820, -79.78646001420200662, 4.059079031676999350 ) ) ;
#29796=ORIENTED_EDGE ( 'NONE', *, *, #19177, .F. ) ;
#29807=CONICAL_SURFACE ( 'NONE', #37370, 11.54999999996000071, 0.7853981633972997312 ) ;
#29818=DIRECTION ( 'NONE',  ( 1.000000000000000000, 0.000000000000000000, 0.000000000000000000 ) ) ;
#29843=CARTESIAN_POINT ( 'NONE',  ( 9.345760913908002010, -78.46240584965400444, 2.683384691900000174 ) ) ;
#29850=ORIENTED_EDGE ( 'NONE', *, *, #52146, .T. ) ;
#29869=DIRECTION ( 'NONE',  ( 1.000000000000000000, 0.000000000000000000, 0.000000000000000000 ) ) ;
#29876=DIRECTION ( 'NONE',  ( 1.044282320439000087E-09, -1.000000000000000000, -6.141137129051000072E-09 ) ) ;
#29885=CARTESIAN_POINT ( 'NONE',  ( 7.184181682494999777, -78.06460333806700191, 6.343145485738000744 ) ) ;
#29904=CARTESIAN_POINT ( 'NONE',  ( -7.662730551410999347, -78.45333667140100431, 6.107448752912000067 ) ) ;
#29911=CARTESIAN_POINT ( 'NONE',  ( 9.500000000000000000, -79.04999999999999716, 0.000000000000000000 ) ) ;
#29943=CARTESIAN_POINT ( 'NONE',  ( -9.500000000000000000, -78.79999999999999716, 0.000000000000000000 ) ) ;
#29956=CARTESIAN_POINT ( 'NONE',  ( 4.335582242278486653, -79.23692256116504495, 8.452722948151309978 ) ) ;
#29959=EDGE_CURVE ( 'NONE', #50093, #53581, #32354, .T. ) ;
#30043=CARTESIAN_POINT ( 'NONE',  ( 9.252740428348992907, -78.67083333333332007, 2.486604901413179025 ) ) ;
#30074=CARTESIAN_POINT ( 'NONE',  ( -8.757268953861998995, -79.72268667140099296, 4.013828826648000003 ) ) ;
#30087=ADVANCED_FACE ( 'NONE', ( #6963 ), #20529, .T. ) ;
#30093=CARTESIAN_POINT ( 'NONE',  ( 8.979348251287998295, -77.90640194988499445, 3.086914251890999772 ) ) ;
#30133=CARTESIAN_POINT ( 'NONE',  ( 4.316051676898999823, -78.96845194988499372, 8.712949996777000550 ) ) ;
#30151=ORIENTED_EDGE ( 'NONE', *, *, #28974, .F. ) ;
#30160=AXIS2_PLACEMENT_3D ( 'NONE', #47344, #6871, #29869 ) ;
#30176=CARTESIAN_POINT ( 'NONE',  ( 9.909302118288000116, -79.00818667140099194, 0.1618955519762999840 ) ) ;
#30189=CARTESIAN_POINT ( 'NONE',  ( 0.000000000000000000, -80.70000000003399521, -9.099999999966000175 ) ) ;
#30221=DIRECTION ( 'NONE',  ( 1.000000000000000000, 0.000000000000000000, 0.000000000000000000 ) ) ;
#30238=CARTESIAN_POINT ( 'NONE',  ( -5.838193839761721016, -78.72708333333332575, 7.596835002782687418 ) ) ;
#30246=AXIS2_PLACEMENT_3D ( 'NONE', #34570, #51747, #11297 ) ;
#30248=EDGE_LOOP ( 'NONE', ( #15339, #28077, #13555 ) ) ;
#30250=CARTESIAN_POINT ( 'NONE',  ( 1.480533219823060742, -79.26251219753629584, 9.383902645560738165 ) ) ;
#30253=ORIENTED_EDGE ( 'NONE', *, *, #16713, .T. ) ;
#30277=EDGE_CURVE ( 'NONE', #12545, #15664, #44683, .T. ) ;
#30278=DIRECTION ( 'NONE',  ( -1.000000000000000000, 0.000000000000000000, 0.000000000000000000 ) ) ;
#30282=CARTESIAN_POINT ( 'NONE',  ( -1.390809606518046193, -79.01333333333329279, -9.431280820568582968 ) ) ;
#30288=ORIENTED_EDGE ( 'NONE', *, *, #3957, .F. ) ;
#30290=CARTESIAN_POINT ( 'NONE',  ( -1.000000000000000000, -75.20000000000000284, 7.200000000000000178 ) ) ;
#30323=CARTESIAN_POINT ( 'NONE',  ( 9.468750000004000356, -79.53124999999600675, -6.681056941828999630E-10 ) ) ;
#30329=CARTESIAN_POINT ( 'NONE',  ( 9.872661273383000591, -77.07106001420200414, 0.04965331886949000267 ) ) ;
#30337=ADVANCED_FACE ( 'NONE', ( #27798, #41102 ), #35782, .F. ) ;
#30355=CYLINDRICAL_SURFACE ( 'NONE', #311, 9.199999999999999289 ) ;
#30384=ORIENTED_EDGE ( 'NONE', *, *, #1306, .T. ) ;
#30419=EDGE_CURVE ( 'NONE', #233, #37512, #33698, .T. ) ;
#30427=CARTESIAN_POINT ( 'NONE',  ( 2.210712544800999879, -79.21319805011499682, -9.468498208576999531 ) ) ;
#30468=EDGE_CURVE ( 'NONE', #10884, #22005, #34717, .T. ) ;
#30474=CARTESIAN_POINT ( 'NONE',  ( 8.072669757012000957, -78.05008667140099021, 4.870514429535999668 ) ) ;
#30477=EDGE_LOOP ( 'NONE', ( #56621, #4023, #50318, #55034 ) ) ;
#30483=CARTESIAN_POINT ( 'NONE',  ( -5.033129434213242881, -79.48027501432439124, -8.057022635265637334 ) ) ;
#30513=AXIS2_PLACEMENT_3D ( 'NONE', #14459, #42504, #46367 ) ;
#30522=CARTESIAN_POINT ( 'NONE',  ( 4.067416459488999436, -79.17074415034599610, -8.418325902196000854 ) ) ;
#30541=AXIS2_PLACEMENT_3D ( 'NONE', #14135, #37448, #55466 ) ;
#30543=CARTESIAN_POINT ( 'NONE',  ( -6.268809852910352198, -79.33229580225618349, 7.139848268590238689 ) ) ;
#30622=CARTESIAN_POINT ( 'NONE',  ( 8.835761575230000275, -77.10746001420200457, 4.404575387497999372 ) ) ;
#30640=ORIENTED_EDGE ( 'NONE', *, *, #19222, .F. ) ;
#30653=CARTESIAN_POINT ( 'NONE',  ( 3.082700750924999955, -79.47186001420199375, -9.022326502593001507 ) ) ;
#30672=CARTESIAN_POINT ( 'NONE',  ( 5.102724688570000389, -78.01904751632000057, 7.811319209985999379 ) ) ;
#30690=DIRECTION ( 'NONE',  ( 1.000000000000000000, 0.000000000000000000, 0.000000000000000000 ) ) ;
#30705=CARTESIAN_POINT ( 'NONE',  ( 4.470112180701956817, -77.00000000000000000, 8.126903283748925233 ) ) ;
#30707=CARTESIAN_POINT ( 'NONE',  ( 0.000000000000000000, -79.50000000000000000, 0.000000000000000000 ) ) ;
#30708=CARTESIAN_POINT ( 'NONE',  ( 7.048436826466999428, -77.99787251632000107, 6.223291978577000449 ) ) ;
#30729=B_SPLINE_CURVE_WITH_KNOTS ( 'NONE', 3,
 ( #12532, #20533, #16683, #34379, #48562, #38531, #52124, #24955, #25530, #34665, #7531, #44126, #30238, #8106, #16392, #12814, #52410, #29943 ),
 .UNSPECIFIED., .F., .F.,
 ( 4, 2, 2, 2, 2, 2, 2, 2, 4 ),
 ( 0.000000000000000000, 0.1250000000000000278, 0.2500000000000000555, 0.3750000000000001110, 0.5000000000000001110, 0.6250000000000001110, 0.7500000000000002220, 0.8750000000000001110, 1.000000000000000000 ),
 .UNSPECIFIED. ) ;
#30751=CARTESIAN_POINT ( 'NONE',  ( -0.6447613848864999220, -78.00963998579798897, 9.665783406873000416 ) ) ;
#30760=CARTESIAN_POINT ( 'NONE',  ( -9.500000000000000000, -78.89999999999999147, 0.000000000000000000 ) ) ;
#30762=CARTESIAN_POINT ( 'NONE',  ( -2.935661446561999899, -79.50000000000000000, -9.035036904803998681 ) ) ;
#30776=CARTESIAN_POINT ( 'NONE',  ( 0.000000000000000000, -75.20000000000000284, -7.200000000000000178 ) ) ;
#30777=ADVANCED_FACE ( 'NONE', ( #705 ), #18393, .F. ) ;
#30798=CARTESIAN_POINT ( 'NONE',  ( 0.000000000000000000, -75.00000000000000000, -7.200000000000000178 ) ) ;
#30813=CYLINDRICAL_SURFACE ( 'NONE', #33065, 9.500000000000000000 ) ;
#30827=CARTESIAN_POINT ( 'NONE',  ( -3.634880433973583180, -79.30591575590990772, 8.776894603130271477 ) ) ;
#30831=AXIS2_PLACEMENT_3D ( 'NONE', #50704, #28225, #42709 ) ;
#30905=CARTESIAN_POINT ( 'NONE',  ( -1.296582552281000167, -77.37128667140099481, -9.676207389328999042 ) ) ;
#30911=CARTESIAN_POINT ( 'NONE',  ( 1.199999999999999956, -75.00000000000000000, -7.200000000000000178 ) ) ;
#30929=DIRECTION ( 'NONE',  ( 0.000000000000000000, -1.000000000000000000, 0.000000000000000000 ) ) ;
#30933=CYLINDRICAL_SURFACE ( 'NONE', #19873, 9.500000000000000000 ) ;
#30951=ORIENTED_EDGE ( 'NONE', *, *, #23726, .T. ) ;
#30974=CONICAL_SURFACE ( 'NONE', #20643, 5.599999999950999729, 0.2449786631268792425 ) ;
#30979=CARTESIAN_POINT ( 'NONE',  ( -4.504865641233999796, -77.29261498579799650, 8.632419597676001644 ) ) ;
#30990=CARTESIAN_POINT ( 'NONE',  ( 0.000000000000000000, -79.65000000003199432, -9.349999999968000353 ) ) ;
#30994=CARTESIAN_POINT ( 'NONE',  ( -3.230363664242999810, -78.10789415034599870, -9.171071524558000121 ) ) ;
#31035=AXIS2_PLACEMENT_3D ( 'NONE', #35330, #53357, #44500 ) ;
#31036=CARTESIAN_POINT ( 'NONE',  ( -5.743104117080999771, -79.05483998579799731, 7.801152530868000312 ) ) ;
#31044=CARTESIAN_POINT ( 'NONE',  ( -9.252740428349001789, -77.42083333333333428, -2.486604901413163926 ) ) ;
#31048=CARTESIAN_POINT ( 'NONE',  ( -6.759806091175823539, -79.46177246518648474, -6.674805502530112733 ) ) ;
#31054=CARTESIAN_POINT ( 'NONE',  ( -2.485321053156992477, -79.19615742320637253, 9.250752650985239356 ) ) ;
#31067=LINE ( 'NONE', #8655, #8136 ) ;
#31074=EDGE_CURVE ( 'NONE', #18799, #34669, #39580, .T. ) ;
#31079=CIRCLE ( 'NONE', #35815, 9.199999999999999289 ) ;
#31084=EDGE_CURVE ( 'NONE', #35308, #15664, #3857, .T. ) ;
#31103=ORIENTED_EDGE ( 'NONE', *, *, #39099, .T. ) ;
#31108=CARTESIAN_POINT ( 'NONE',  ( 1.400971506258957167, -79.26317057520080311, 9.396169613821864885 ) ) ;
#31114=CARTESIAN_POINT ( 'NONE',  ( 6.668756384172233709, -79.48666666666666458, -6.812569087104355603 ) ) ;
#31115=EDGE_CURVE ( 'NONE', #3607, #42830, #50230, .T. ) ;
#31125=CARTESIAN_POINT ( 'NONE',  ( 6.220862042517180335, -77.86622231854060772, 6.858636509587040742 ) ) ;
#31143=CARTESIAN_POINT ( 'NONE',  ( -2.335995526795000110, -79.61238667140099778, -9.341389049788000776 ) ) ;
#31193=CARTESIAN_POINT ( 'NONE',  ( 3.145085892150000006, -77.47146001420199468, -9.358399194681000566 ) ) ;
#31196=CARTESIAN_POINT ( 'NONE',  ( -9.500000000000000000, -78.79999999999999716, 0.000000000000000000 ) ) ;
#31200=CARTESIAN_POINT ( 'NONE',  ( 8.395992668097999712, -79.43960095943374711, 4.560928606276999808 ) ) ;
#31229=CARTESIAN_POINT ( 'NONE',  ( -1.863129461298999923, -79.73813998579800000, -9.025265489830999854 ) ) ;
#31238=VERTEX_POINT ( 'NONE', #18028 ) ;
#31249=CARTESIAN_POINT ( 'NONE',  ( -2.712012240502000182, -77.58820584965398837, 9.099584490865000319 ) ) ;
#31268=CARTESIAN_POINT ( 'NONE',  ( 0.000000000000000000, -78.00000000000000000, -7.200000000000000178 ) ) ;
#31270=CARTESIAN_POINT ( 'NONE',  ( 1.761422869556999782, -77.51881498579798802, -9.576527127505000792 ) ) ;
#31276=ORIENTED_EDGE ( 'NONE', *, *, #43462, .F. ) ;
#31285=CARTESIAN_POINT ( 'NONE',  ( -5.600962501326000265, -77.93369415034599967, 7.948110234177999445 ) ) ;
#31319=CARTESIAN_POINT ( 'NONE',  ( 1.243547092045969915, -78.53541666666666288, -9.500000000000000000 ) ) ;
#31342=CARTESIAN_POINT ( 'NONE',  ( -8.475401746435078820, -79.43728386678893116, -4.291540307597959902 ) ) ;
#31343=LINE ( 'NONE', #4212, #35540 ) ;
#31360=CARTESIAN_POINT ( 'NONE',  ( 9.252740428349003565, -78.52916666666668277, -2.486604901413146607 ) ) ;
#31411=CARTESIAN_POINT ( 'NONE',  ( 1.224189701827945287, -79.26463158461723424, 9.420864478166739886 ) ) ;
#31425=CARTESIAN_POINT ( 'NONE',  ( 7.324086682717548591, -77.85317212802200970, 5.812447148214148207 ) ) ;
#31428=CARTESIAN_POINT ( 'NONE',  ( 0.6604400869868999324, -77.13741167140099719, -9.497136025460999775 ) ) ;
#31474=ORIENTED_EDGE ( 'NONE', *, *, #31836, .F. ) ;
#31478=CARTESIAN_POINT ( 'NONE',  ( 0.000000000000000000, -75.20000000000000284, 6.200000000000000178 ) ) ;
#31490=CARTESIAN_POINT ( 'NONE',  ( 7.443337284218999983, -78.06288667140100301, 6.317073012428999768 ) ) ;
#31497=CARTESIAN_POINT ( 'NONE',  ( 3.938458446976999205, -79.30999999999998806, -8.369650235310999165 ) ) ;
#31526=CARTESIAN_POINT ( 'NONE',  ( -9.501130936298000762, -79.68751332859899605, 0.6697165097470000328 ) ) ;
#31528=ADVANCED_FACE ( 'NONE', ( #38396 ), #55837, .T. ) ;
#31548=CARTESIAN_POINT ( 'NONE',  ( 3.861138328465000047, -76.97116028321799774, 8.493887087553000370 ) ) ;
#31566=CARTESIAN_POINT ( 'NONE',  ( -9.104587144006000443, -77.46948832859899881, -3.133183417595999831 ) ) ;
#31580=CARTESIAN_POINT ( 'NONE',  ( -8.871933854994999535, -78.60349805011500735, -3.979018739998999354 ) ) ;
#31594=DIRECTION ( 'NONE',  ( 1.000000000000000000, 0.000000000000000000, 0.000000000000000000 ) ) ;
#31618=CARTESIAN_POINT ( 'NONE',  ( 9.500000000000000000, -78.64999999999999147, 0.000000000000000000 ) ) ;
#31626=CARTESIAN_POINT ( 'NONE',  ( -5.485200302047999799, -78.70643998579799927, -7.984597978739000901 ) ) ;
#31635=DIRECTION ( 'NONE',  ( 0.000000000000000000, 1.000000000000000000, 7.261213190611999915E-14 ) ) ;
#31638=CARTESIAN_POINT ( 'NONE',  ( -9.034242263150824570, -79.42472277150091031, -2.937518930512160509 ) ) ;
#31659=ORIENTED_EDGE ( 'NONE', *, *, #7385, .T. ) ;
#31662=CARTESIAN_POINT ( 'NONE',  ( -6.013262726775999489, -77.57957403538303254, 7.348341287529000176 ) ) ;
#31666=CARTESIAN_POINT ( 'NONE',  ( 9.500000000000005329, -77.53958333333333997, -1.243547092045939939 ) ) ;
#31739=CARTESIAN_POINT ( 'NONE',  ( 1.807226454530999948, -79.43046001420199786, 9.346133917991000573 ) ) ;
#31740=DIRECTION ( 'NONE',  ( -1.000000000000000000, 0.000000000000000000, 0.000000000000000000 ) ) ;
#31756=VERTEX_POINT ( 'NONE', #23588 ) ;
#31789=DIRECTION ( 'NONE',  ( 0.000000000000000000, 1.000000000000000000, 0.000000000000000000 ) ) ;
#31792=CARTESIAN_POINT ( 'NONE',  ( 4.324825231101488754, -77.06249999999998579, -8.491324637162149358 ) ) ;
#31823=CARTESIAN_POINT ( 'NONE',  ( 6.055527902613000002, -78.11999999999999034, 7.319875806370000682 ) ) ;
#31828=CARTESIAN_POINT ( 'NONE',  ( 8.000597322312000159, -79.42353998579800134, 4.965221403244999721 ) ) ;
#31836=EDGE_CURVE ( 'NONE', #41593, #15380, #53095, .T. ) ;
#31847=CARTESIAN_POINT ( 'NONE',  ( -8.383077572658999443, -77.59115194988500264, 4.458862939031999595 ) ) ;
#31866=CARTESIAN_POINT ( 'NONE',  ( -7.146006657343000334, -77.38466332859900376, 6.453288637825999707 ) ) ;
#31877=CARTESIAN_POINT ( 'NONE',  ( 4.316051676898999823, -78.90834805011499498, 8.712949996777000550 ) ) ;
#31891=VERTEX_POINT ( 'NONE', #52211 ) ;
#31910=CARTESIAN_POINT ( 'NONE',  ( -8.300970689365447797, -78.44166666666664867, -4.784380313523547201 ) ) ;
#31921=CARTESIAN_POINT ( 'NONE',  ( -6.090801878186413276, -79.47970282387936436, 7.362514718212188392 ) ) ;
#31930=CONICAL_SURFACE ( 'NONE', #13097, 1.099999997158000120, 0.7853981633972997312 ) ;
#31979=CIRCLE ( 'NONE', #31035, 5.100000000000000533 ) ;
#31993=EDGE_CURVE ( 'NONE', #13771, #51311, #46121, .T. ) ;
#32015=CARTESIAN_POINT ( 'NONE',  ( -9.067070616629999691, -78.97593667140100138, 3.715721191563000403 ) ) ;
#32032=CARTESIAN_POINT ( 'NONE',  ( -8.697106840384998705, -79.54218667140099797, -4.132666167052000183 ) ) ;
#32048=DIRECTION ( 'NONE',  ( 0.000000000000000000, 1.000000000000000000, 0.000000000000000000 ) ) ;
#32064=CARTESIAN_POINT ( 'NONE',  ( 9.425400508419963685, -79.15997041332948925, 1.202743096264716982 ) ) ;
#32087=CARTESIAN_POINT ( 'NONE',  ( -9.299222834567000717, -77.67151332859899071, 2.587993818716000316 ) ) ;
#32119=CARTESIAN_POINT ( 'NONE',  ( 8.158537514794998557, -79.33773998579800946, -4.701213835425000376 ) ) ;
#32126=DIRECTION ( 'NONE',  ( 0.000000000000000000, 1.000000000000000000, 0.000000000000000000 ) ) ;
#32132=EDGE_LOOP ( 'NONE', ( #8404, #23323, #38637, #34534 ) ) ;
#32138=CARTESIAN_POINT ( 'NONE',  ( -8.123853732960998997, -77.02664805011499993, 4.915330883505999893 ) ) ;
#32147=CARTESIAN_POINT ( 'NONE',  ( 7.596835002782697188, -77.60208333333335418, 5.838193839761710358 ) ) ;
#32156=CARTESIAN_POINT ( 'NONE',  ( 5.344729029608000559, -77.70731498579799279, 7.975868177029001416 ) ) ;
#32165=CARTESIAN_POINT ( 'NONE',  ( 6.233080334754680152, -77.00000000000000000, 6.909364586181893308 ) ) ;
#32199=CARTESIAN_POINT ( 'NONE',  ( -4.855043705795098141, -77.81750000000000966, 8.214633846514278304 ) ) ;
#32210=CARTESIAN_POINT ( 'NONE',  ( 1.924380748938630393E-07, -79.75000000000001421, -9.249538042332323684 ) ) ;
#32253=EDGE_CURVE ( 'NONE', #39245, #22854, #13490, .T. ) ;
#32264=CARTESIAN_POINT ( 'NONE',  ( -1.243547092045951041, -77.91458333333331154, -9.500000000000000000 ) ) ;
#32293=CARTESIAN_POINT ( 'NONE',  ( 6.644230831661016801, -77.23692193750341062, -6.715582363013730571 ) ) ;
#32299=CARTESIAN_POINT ( 'NONE',  ( 4.349579488465999511, -78.84528667140098435, 8.780633650160998727 ) ) ;
#32304=DIRECTION ( 'NONE',  ( -1.000000000000000000, 0.000000000000000000, 0.000000000000000000 ) ) ;
#32317=CARTESIAN_POINT ( 'NONE',  ( 9.027693294681998992, -79.16251332859900458, -3.653265801962000126 ) ) ;
#32336=ORIENTED_EDGE ( 'NONE', *, *, #11339, .T. ) ;
#32354=LINE ( 'NONE', #10235, #41250 ) ;
#32373=CARTESIAN_POINT ( 'NONE',  ( 5.848847972528999684, -77.01631332859899715, 7.678821120301999592 ) ) ;
#32376=CARTESIAN_POINT ( 'NONE',  ( 6.739285134038754066, -77.08750000000004832, -6.737116835514523672 ) ) ;
#32402=CARTESIAN_POINT ( 'NONE',  ( 1.930387568569762236, -77.00000000000001421, 9.098804631813305122 ) ) ;
#32406=CARTESIAN_POINT ( 'NONE',  ( 8.252635040182997983, -79.40151332859900890, -4.755435880420999517 ) ) ;
#32408=ORIENTED_EDGE ( 'NONE', *, *, #31836, .T. ) ;
#32425=CARTESIAN_POINT ( 'NONE',  ( 1.529609450199000076, -76.93207305011499386, 9.371081266747001592 ) ) ;
#32434=CARTESIAN_POINT ( 'NONE',  ( -9.500000000000007105, -77.78958333333335418, 1.243547092045919733 ) ) ;
#32452=CARTESIAN_POINT ( 'NONE',  ( 8.689834030816680155, -76.99999999999998579, 3.513648003987066115 ) ) ;
#32480=CARTESIAN_POINT ( 'NONE',  ( -3.300471783580745999, -77.00000000000002842, -8.910846386529984287 ) ) ;
#32488=CARTESIAN_POINT ( 'NONE',  ( -3.234762833941022819, -77.80249999999999488, 8.977080150340215781 ) ) ;
#32533=CARTESIAN_POINT ( 'NONE',  ( 1.009320482739999969, -77.51652403538301428, 9.441330439200999791 ) ) ;
#32571=CARTESIAN_POINT ( 'NONE',  ( 9.665471083832999355, -78.54936001420199432, -2.650702293911000318 ) ) ;
#32588=CARTESIAN_POINT ( 'NONE',  ( 5.216320339343518242, -77.37829693750339288, 7.876220663163953972 ) ) ;
#32618=CARTESIAN_POINT ( 'NONE',  ( 4.067416459488999436, -79.35105584965398862, -8.418325902196000854 ) ) ;
#32652=PLANE ( 'NONE',  #30831 ) ;
#32663=CARTESIAN_POINT ( 'NONE',  ( 4.980329458316080427, -77.06875000000002274, -8.124224631303468058 ) ) ;
#32673=AXIS2_PLACEMENT_3D ( 'NONE', #38444, #46756, #16015 ) ;
#32682=EDGE_CURVE ( 'NONE', #16336, #34323, #42548, .T. ) ;
#32715=CARTESIAN_POINT ( 'NONE',  ( 5.102724688570000389, -77.89883971678199259, 7.811319209985999379 ) ) ;
#32734=EDGE_CURVE ( 'NONE', #45676, #3012, #24407, .T. ) ;
#32735=CARTESIAN_POINT ( 'NONE',  ( -6.314216249843999762, -76.81193998579799143, 7.143954968317999921 ) ) ;
#32739=ORIENTED_EDGE ( 'NONE', *, *, #27863, .T. ) ;
#32743=LINE ( 'NONE', #50791, #16304 ) ;
#32771=CARTESIAN_POINT ( 'NONE',  ( -6.507505845087319329, -76.99999999999998579, -6.850455418477346292 ) ) ;
#32777=CARTESIAN_POINT ( 'NONE',  ( -6.933189095244579825, -79.72395833333175119, -6.238628562272925393 ) ) ;
#32780=CARTESIAN_POINT ( 'NONE',  ( 2.278690965393999956, -79.02258998579800675, -9.759650287631000509 ) ) ;
#32803=ADVANCED_FACE ( 'NONE', ( #42422 ), #11135, .T. ) ;
#32804=FACE_OUTER_BOUND ( 'NONE', #47781, .T. ) ;
#32809=EDGE_CURVE ( 'NONE', #11254, #11325, #51771, .T. ) ;
#32828=FACE_OUTER_BOUND ( 'NONE', #49664, .T. ) ;
#32834=DIRECTION ( 'NONE',  ( 3.497202527557000183E-12, 1.000000000000000000, 1.787522907329000142E-11 ) ) ;
#32847=CARTESIAN_POINT ( 'NONE',  ( 9.500000000000000000, -77.54999999999999716, 0.000000000000000000 ) ) ;
#32851=CARTESIAN_POINT ( 'NONE',  ( 5.948961716885869500, -78.02087376917042150, 7.191048434022237146 ) ) ;
#32860=VECTOR ( 'NONE', #6239, 1000.000000000000000 ) ;
#32863=CARTESIAN_POINT ( 'NONE',  ( -7.762343146465000565, -78.37516001420199530, -6.339840787406999745 ) ) ;
#32885=CARTESIAN_POINT ( 'NONE',  ( -0.8449659473473000171, -78.95261001420199420, 9.650246712936999316 ) ) ;
#32899=ADVANCED_FACE ( 'NONE', ( #41454 ), #43274, .F. ) ;
#32911=CARTESIAN_POINT ( 'NONE',  ( -9.554796630153999715, -79.57014805011500869, -0.02401403847836000235 ) ) ;
#32957=CARTESIAN_POINT ( 'NONE',  ( 9.438309774439000321, -77.92631332859899373, -2.022706718371000356 ) ) ;
#32960=CARTESIAN_POINT ( 'NONE',  ( -0.001533218590079363447, -77.02500000000000568, -9.529255218666872196 ) ) ;
#32969=CARTESIAN_POINT ( 'NONE',  ( 2.013632425233999879, -78.15144415034599490, -9.512575055159999238 ) ) ;
#32992=ORIENTED_EDGE ( 'NONE', *, *, #1306, .F. ) ;
#33011=CARTESIAN_POINT ( 'NONE',  ( -8.123853732960998997, -76.96654415034599594, 4.915330883505999893 ) ) ;
#33063=DIRECTION ( 'NONE',  ( 1.000000000000000000, 0.000000000000000000, 0.000000000000000000 ) ) ;
#33065=AXIS2_PLACEMENT_3D ( 'NONE', #3394, #48845, #52411 ) ;
#33155=AXIS2_PLACEMENT_3D ( 'NONE', #14412, #10008, #40711 ) ;
#33172=CARTESIAN_POINT ( 'NONE',  ( 1.924380748938630393E-07, -79.75000000000001421, -9.249538042332323684 ) ) ;
#33174=CARTESIAN_POINT ( 'NONE',  ( 0.6553672983243258310, -77.18037193750340919, -9.424189266312801294 ) ) ;
#33177=CARTESIAN_POINT ( 'NONE',  ( -5.743104117080999771, -78.99616001420199041, 7.801152530868000312 ) ) ;
#33205=CARTESIAN_POINT ( 'NONE',  ( 8.150225256662000817, -79.90095584965399667, -4.374508917085999649 ) ) ;
#33226=CARTESIAN_POINT ( 'NONE',  ( 4.403238962115728405, -79.23630107778137699, 8.417739988564747478 ) ) ;
#33247=CARTESIAN_POINT ( 'NONE',  ( -8.742972704348000335, -77.54048501420199102, 3.483847966513999861 ) ) ;
#33250=CARTESIAN_POINT ( 'NONE',  ( -1.243547092045992564, -77.18541666666664014, 9.499999999999994671 ) ) ;
#33263=CARTESIAN_POINT ( 'NONE',  ( 3.973905474789803716, -79.36013131668573806, -8.444981681530821405 ) ) ;
#33279=AXIS2_PLACEMENT_3D ( 'NONE', #7633, #15921, #55793 ) ;
#33298=ORIENTED_EDGE ( 'NONE', *, *, #40025, .F. ) ;
#33315=CARTESIAN_POINT ( 'NONE',  ( -9.603246065258371544, -79.06172913613842468, -1.533382312990622998 ) ) ;
#33326=CARTESIAN_POINT ( 'NONE',  ( 8.300970689365442468, -78.69166666666666288, 4.784380313523563188 ) ) ;
#33375=CARTESIAN_POINT ( 'NONE',  ( -7.762343146465000565, -77.93383998579800220, -6.339840787406999745 ) ) ;
#33380=CARTESIAN_POINT ( 'NONE',  ( -9.018298289885381180, -79.37428396167247513, 2.986588901158017784 ) ) ;
#33434=EDGE_CURVE ( 'NONE', #23500, #23213, #13593, .T. ) ;
#33451=ORIENTED_EDGE ( 'NONE', *, *, #27793, .F. ) ;
#33457=CARTESIAN_POINT ( 'NONE',  ( 4.739769873023999658, -78.98486001420198477, -8.830749431300999319 ) ) ;
#33464=CARTESIAN_POINT ( 'NONE',  ( 6.055527902613000002, -77.71999999999999886, 7.319875806370000682 ) ) ;
#33475=CARTESIAN_POINT ( 'NONE',  ( -5.611728806388999402, -78.52021332859899871, -8.168780722191000265 ) ) ;
#33489=AXIS2_PLACEMENT_3D ( 'NONE', #3094, #56824, #16670 ) ;
#33498=CARTESIAN_POINT ( 'NONE',  ( -6.169975633831000117, -79.51351332859900367, -7.535017646125999669 ) ) ;
#33503=CARTESIAN_POINT ( 'NONE',  ( 5.395043866960259393, -77.97557524174651178, 7.539927916798925267 ) ) ;
#33517=FACE_OUTER_BOUND ( 'NONE', #30477, .T. ) ;
#33525=CARTESIAN_POINT ( 'NONE',  ( 9.036425267681602591, -79.17454650634799407, 2.930576671598891014 ) ) ;
#33551=DIRECTION ( 'NONE',  ( 0.000000000000000000, 0.000000000000000000, -1.000000000000000000 ) ) ;
#33597=ORIENTED_EDGE ( 'NONE', *, *, #15132, .F. ) ;
#33602=CARTESIAN_POINT ( 'NONE',  ( 8.979348251287998295, -77.78619415034600593, 3.086914251890999772 ) ) ;
#33606=CARTESIAN_POINT ( 'NONE',  ( 4.316728918958533612, -78.88752913613843987, 8.714317166737037823 ) ) ;
#33613=CARTESIAN_POINT ( 'NONE',  ( -2.486604901413153268, -78.00416666666664867, -9.252740428348998236 ) ) ;
#33653=CARTESIAN_POINT ( 'NONE',  ( -9.126674389914770202, -76.99999999999998579, 1.824525243212377523 ) ) ;
#33665=AXIS2_PLACEMENT_3D ( 'NONE', #29343, #47683, #16077 ) ;
#33689=SURFACE_SIDE_STYLE ('',( #15986 ) ) ;
#33698=CIRCLE ( 'NONE', #17688, 1.000000000000000000 ) ;
#33711=CARTESIAN_POINT ( 'NONE',  ( 0.000000000000000000, -75.00000000000000000, 7.200000000000000178 ) ) ;
#33719=CARTESIAN_POINT ( 'NONE',  ( 11.65000000000000036, -76.00000000000000000, 0.000000000000000000 ) ) ;
#33748=CARTESIAN_POINT ( 'NONE',  ( -9.067070616629999691, -79.16216332859900717, 3.715721191563000403 ) ) ;
#33764=CARTESIAN_POINT ( 'NONE',  ( 5.381001269034999979, -79.11539666193300491, -7.930497238065998822 ) ) ;
#33772=CYLINDRICAL_SURFACE ( 'NONE', #33665, 9.500000000000000000 ) ;
#33774=ORIENTED_EDGE ( 'NONE', *, *, #16691, .T. ) ;
#33789=CARTESIAN_POINT ( 'NONE',  ( -5.764562846862999912, -79.07549514476063734, 7.830301022820999712 ) ) ;
#33792=CARTESIAN_POINT ( 'NONE',  ( -8.650571159592999493, -79.47494415034599058, 4.057379972786000266 ) ) ;
#33810=CARTESIAN_POINT ( 'NONE',  ( 8.810121547015370425, -79.18024560760937902, 3.560590676149650413 ) ) ;
#33812=DIRECTION ( 'NONE',  ( 0.000000000000000000, 1.000000000000000000, 0.000000000000000000 ) ) ;
#33829=CARTESIAN_POINT ( 'NONE',  ( -8.843810886990000952, -77.47671167140099158, 3.524029368129000250 ) ) ;
#33842=CARTESIAN_POINT ( 'NONE',  ( -2.486604901413195901, -78.29583333333336270, 9.252740428348989354 ) ) ;
#33882=ADVANCED_FACE ( 'NONE', ( #50713 ), #50455, .T. ) ;
#33885=CARTESIAN_POINT ( 'NONE',  ( -6.013262726775999489, -77.43941915034599788, 7.348341287529000176 ) ) ;
#33888=CARTESIAN_POINT ( 'NONE',  ( 5.395886906468551736, -77.87470926922809156, 7.541113365569439786 ) ) ;
#33954=VECTOR ( 'NONE', #23545, 1000.000000000000000 ) ;
#33963=CARTESIAN_POINT ( 'NONE',  ( 0.000000000000000000, -75.00000000000000000, 0.000000000000000000 ) ) ;
#33975=CARTESIAN_POINT ( 'NONE',  ( 7.090970028742000331, -77.75223832859899176, 6.513691531324999673 ) ) ;
#34030=CARTESIAN_POINT ( 'NONE',  ( -5.809342935555999787, -79.11861332859899676, 7.891128111295000025 ) ) ;
#34033=ORIENTED_EDGE ( 'NONE', *, *, #16238, .T. ) ;
#34036=CARTESIAN_POINT ( 'NONE',  ( 9.499999999999998224, -77.66166666666666174, 1.392772743091435617 ) ) ;
#34048=CARTESIAN_POINT ( 'NONE',  ( -3.403932870613000095, -78.34601332859899969, 9.307723658127001087 ) ) ;
#34054=CARTESIAN_POINT ( 'NONE',  ( 8.300970689365456678, -79.00833333333333997, -4.784380313523530326 ) ) ;
#34080=CARTESIAN_POINT ( 'NONE',  ( 1.861092857305999937, -79.65044415034600434, -9.371850619045000386 ) ) ;
#34092=ORIENTED_EDGE ( 'NONE', *, *, #9937, .F. ) ;
#34095=CARTESIAN_POINT ( 'NONE',  ( 4.321906625261624946, -79.23704788471283678, 8.459721384812338485 ) ) ;
#34113=CARTESIAN_POINT ( 'NONE',  ( -7.596835002782738933, -77.24791666666669698, 5.838193839761661508 ) ) ;
#34146=VERTEX_POINT ( 'NONE', #48519 ) ;
#34169=CARTESIAN_POINT ( 'NONE',  ( 3.861138328465000047, -76.91105638344899376, 8.493887087553000370 ) ) ;
#34181=CARTESIAN_POINT ( 'NONE',  ( 9.653543233641000754, -78.05386001420200159, -2.068833003092999778 ) ) ;
#34202=DIRECTION ( 'NONE',  ( 0.000000000000000000, 1.000000000000000000, 0.000000000000000000 ) ) ;
#34224=CARTESIAN_POINT ( 'NONE',  ( -8.216989605509789740, -77.00000000000000000, 4.339777185649433378 ) ) ;
#34227=CARTESIAN_POINT ( 'NONE',  ( -5.100000000000000533, -75.20000000000000284, 0.000000000000000000 ) ) ;
#34242=CONICAL_SURFACE ( 'NONE', #29289, 9.099999999966000175, 0.7853981633972997312 ) ;
#34275=CARTESIAN_POINT ( 'NONE',  ( 1.899930039692999895, -78.48940194988499286, 9.535935523283001203 ) ) ;
#34319=CARTESIAN_POINT ( 'NONE',  ( 9.449971683680001178, -78.42181332859900067, -2.591602768458999950 ) ) ;
#34323=VERTEX_POINT ( 'NONE', #343 ) ;
#34338=CARTESIAN_POINT ( 'NONE',  ( -9.170454433240001535, -78.91216332859900717, 3.758088286126999744 ) ) ;
#34349=LINE ( 'NONE', #51814, #26316 ) ;
#34379=CARTESIAN_POINT ( 'NONE',  ( 8.300970689365438915, -78.59166666666666856, 4.784380313523563188 ) ) ;
#34389=CARTESIAN_POINT ( 'NONE',  ( 3.858042142442956735, -79.24129547567945053, 8.682305691183742624 ) ) ;
#34395=CARTESIAN_POINT ( 'NONE',  ( -9.555308244098332793, -79.54990282387937839, -0.02401532431606494614 ) ) ;
#34405=AXIS2_PLACEMENT_3D ( 'NONE', #55069, #41787, #42378 ) ;
#34420=CARTESIAN_POINT ( 'NONE',  ( -5.838193839761721016, -78.32708333333332007, 7.596835002782687418 ) ) ;
#34463=CARTESIAN_POINT ( 'NONE',  ( 6.670495747569742839, -78.23427913613843998, -7.076578245536430778 ) ) ;
#34469=CARTESIAN_POINT ( 'NONE',  ( -6.380837375266275480, -79.36735876298251924, -7.083146235777555866 ) ) ;
#34470=CARTESIAN_POINT ( 'NONE',  ( 7.527250314086999516, -78.12666001420200246, 6.388289016235000339 ) ) ;
#34474=CARTESIAN_POINT ( 'NONE',  ( 9.500000000000000000, -78.64999999999999147, 0.000000000000000000 ) ) ;
#34505=CARTESIAN_POINT ( 'NONE',  ( -1.927595379902999895, -79.92946001420199309, -9.337547616506999049 ) ) ;
#34510=CARTESIAN_POINT ( 'NONE',  ( -9.131943537062705119, -77.00000000000000000, 1.799860230811830997 ) ) ;
#34522=CARTESIAN_POINT ( 'NONE',  ( 3.861138328465000047, -77.03126418298700173, 8.493887087553000370 ) ) ;
#34534=ORIENTED_EDGE ( 'NONE', *, *, #53369, .F. ) ;
#34536=ORIENTED_EDGE ( 'NONE', *, *, #32809, .T. ) ;
#34553=CARTESIAN_POINT ( 'NONE',  ( -9.312500000004000356, -79.68749999999599254, 6.570867420027000168E-10 ) ) ;
#34563=CARTESIAN_POINT ( 'NONE',  ( -0.6471704932797999188, -78.01035194988499200, 9.701898969124000516 ) ) ;
#34566=CARTESIAN_POINT ( 'NONE',  ( -9.500000000000000000, -78.89999999999999147, 0.000000000000000000 ) ) ;
#34570=CARTESIAN_POINT ( 'NONE',  ( 0.000000000000000000, -76.79999999999999716, 0.000000000000000000 ) ) ;
#34593=AXIS2_PLACEMENT_3D ( 'NONE', #55080, #50671, #50377 ) ;
#34596=DIRECTION ( 'NONE',  ( -1.000000000000000000, 0.000000000000000000, 0.000000000000000000 ) ) ;
#34607=CARTESIAN_POINT ( 'NONE',  ( -9.090572324265000503, -78.22428667140098923, 3.947417077667999763 ) ) ;
#34611=VERTEX_POINT ( 'NONE', #35505 ) ;
#34634=CARTESIAN_POINT ( 'NONE',  ( -9.252740428348994683, -78.82083333333329733, -2.486604901413163926 ) ) ;
#34658=CARTESIAN_POINT ( 'NONE',  ( 7.507056363060000237, -79.70894415034599945, -5.572808305725000189 ) ) ;
#34661=EDGE_CURVE ( 'NONE', #31891, #3607, #6458, .T. ) ;
#34665=CARTESIAN_POINT ( 'NONE',  ( -1.243547092045992564, -78.68541666666664014, 9.499999999999994671 ) ) ;
#34669=VERTEX_POINT ( 'NONE', #14247 ) ;
#34671=ORIENTED_EDGE ( 'NONE', *, *, #34661, .T. ) ;
#34677=CARTESIAN_POINT ( 'NONE',  ( -6.771338525271339392, -79.33792608965413251, 6.663214335040369640 ) ) ;
#34712=LINE ( 'NONE', #56596, #36707 ) ;
#34717=B_SPLINE_CURVE_WITH_KNOTS ( 'NONE', 3,
 ( #36956, #23089, #44953, #49085, #4508, #22209, #22510, #40520, #113, #34469, #52217, #10394, #11493, #2910, #23957, #3205, #15909 ),
 .UNSPECIFIED., .F., .F.,
 ( 4, 2, 1, 2, 2, 2, 2, 2, 4 ),
 ( 0.000000000000000000, 0.04878227772541878643, 0.09756455545083757286, 0.1463468331762563523, 0.1951291109016751457, 0.2439113886270939391, 0.2926936663525128157, 0.3414759440779315813, 0.3902582218033504580 ),
 .UNSPECIFIED. ) ;
#34805=CARTESIAN_POINT ( 'NONE',  ( 0.000000000000000000, -75.20000000000000284, 0.000000000000000000 ) ) ;
#34810=ORIENTED_EDGE ( 'NONE', *, *, #9937, .T. ) ;
#34833=DIRECTION ( 'NONE',  ( 1.000000000000000000, 0.000000000000000000, 0.000000000000000000 ) ) ;
#34848=CARTESIAN_POINT ( 'NONE',  ( 8.219513559211000242, -78.92490194988499752, 5.194554602171000290 ) ) ;
#34876=CIRCLE ( 'NONE', #30160, 6.100000000000000533 ) ;
#34890=ORIENTED_EDGE ( 'NONE', *, *, #17233, .F. ) ;
#34893=CARTESIAN_POINT ( 'NONE',  ( 8.546298008199000762, -78.96463667140099574, -5.018094164374000243 ) ) ;
#34904=CARTESIAN_POINT ( 'NONE',  ( -9.055506177563403369, -79.42412239826263942, -2.871540687672356373 ) ) ;
#34914=CIRCLE ( 'NONE', #83, 1.199999999999999956 ) ;
#34943=CARTESIAN_POINT ( 'NONE',  ( 9.539544502573999551, -79.26434415034600534, 0.5400218831816999687 ) ) ;
#34964=CARTESIAN_POINT ( 'NONE',  ( -6.865937273109800287, -79.33902379046836018, 6.565646674124808513 ) ) ;
#34994=CARTESIAN_POINT ( 'NONE',  ( -9.500000000000001776, -78.90666666666666629, -0.7958701389094111622 ) ) ;
#35011=ORIENTED_EDGE ( 'NONE', *, *, #29687, .T. ) ;
#35034=CARTESIAN_POINT ( 'NONE',  ( 5.790379964274294800, -79.57682291666264973, 7.536004867747862157 ) ) ;
#35041=CARTESIAN_POINT ( 'NONE',  ( -2.575222906043999949, -77.21666001420199166, 9.530972118016000749 ) ) ;
#35074=CARTESIAN_POINT ( 'NONE',  ( 2.846957383478000203, -79.67206001420200323, 9.316630448266000286 ) ) ;
#35082=CARTESIAN_POINT ( 'NONE',  ( -9.500000000000000000, -78.38958333333334849, 1.243547092045920399 ) ) ;
#35091=ORIENTED_EDGE ( 'NONE', *, *, #57860, .T. ) ;
#35096=CARTESIAN_POINT ( 'NONE',  ( 4.001451577097999923, -77.96945194988499850, 8.339717337904000161 ) ) ;
#35099=EDGE_CURVE ( 'NONE', #57123, #23864, #20313, .T. ) ;
#35107=ORIENTED_EDGE ( 'NONE', *, *, #17154, .T. ) ;
#35131=CARTESIAN_POINT ( 'NONE',  ( 4.056922300394875336, -77.00000000000000000, 8.335976438453148063 ) ) ;
#35135=CARTESIAN_POINT ( 'NONE',  ( -0.5312504855272001114, -78.75070194988499850, -9.708839960653000034 ) ) ;
#35141=CARTESIAN_POINT ( 'NONE',  ( -9.372585790538636275, -78.28499999999999659, 1.790612804732440555 ) ) ;
#35164=ORIENTED_EDGE ( 'NONE', *, *, #6182, .T. ) ;
#35175=CARTESIAN_POINT ( 'NONE',  ( 1.892857502466999797, -78.48868998579800405, 9.500437764121999251 ) ) ;
#35186=CARTESIAN_POINT ( 'NONE',  ( -5.510565319487811031, -79.47559583644631687, -7.739628810976011408 ) ) ;
#35202=CARTESIAN_POINT ( 'NONE',  ( -1.243547092045951041, -78.41458333333332575, -9.500000000000000000 ) ) ;
#35206=VERTEX_POINT ( 'NONE', #19941 ) ;
#35214=CARTESIAN_POINT ( 'NONE',  ( 2.486604901413172364, -77.44583333333332575, -9.252740428348998236 ) ) ;
#35240=B_SPLINE_CURVE_WITH_KNOTS ( 'NONE', 3,
 ( #55098, #37374, #10526, #9359, #32064, #50105, #9649, #45679, #5219, #23224, #41228, #18801, #6961, #11120, #33525, #51272, #20545, #46849, #19971, #11404, #33810, #10826, #15822, #1976, #2827, #56556, #16405, #55687, #28802, #51848, #1679, #24965, #47141, #56271, #6378, #20825, #37957, #24681, #25255, #38540, #24392, #29383, #42406, #55981, #47431, #6673, #29097, #2257, #19669, #42693, #16116, #20257, #42984, #33226, #2542, #29956, #34095, #51562, #29669, #48007, #52135, #37668, #34389, #11693, #38830, #11978, #47718, #56847, #7542, #7251, #52420, #43273, #38248, #25541, #15233, #15531, #40287, #58000, #3687, #30250, #8403, #39697, #31108, #52995, #31411, #44139, #21404, #12258, #49149, #26118, #39416, #53878, #35548, #22271, #48576, #3406, #13114, #8700, #12544, #17859, #25830, #26690, #52706, #3124, #44722, #43858, #58298, #13411, #35848, #30827, #21115, #8118, #12827, #57420, #17260, #49454, #16696, #48861, #7830, #4275, #17556, #26400, #35250, #21689, #9000, #43559, #21975, #30543, #44422, #39122, #57129, #48291, #34677, #16982, #34964, #57705, #53281, #3973, #39986, #53577, #50832, #28362, #4573, #49749, #9292, #40585, #26985, #1531, #1246, #46409, #10678, #19525, #5937, #33380, #24534, #6228, #24244, #42546, #42260, #28071, #182, #10377, #55834, #23654, #22573, #2114, #13707, #20113, #38104, #51416, #14790, #56124, #18156, #46994, #54167, #36150, #41959, #46119, #28952 ),
 .UNSPECIFIED., .F., .F.,
 ( 4, 2, 2, 2, 2, 2, 1, 2, 2, 1, 1, 2, 2, 2, 2, 2, 2, 2, 1, 1, 2, 2, 2, 1, 1, 2, 2, 1, 2, 2, 2, 1, 2, 2, 1, 1, 2, 1, 2, 2, 2, 1, 2, 2, 2, 2, 2, 1, 1, 1, 2, 2, 2, 2, 2, 2, 2, 1, 2, 2, 2, 2, 2, 2, 1, 2, 2, 2, 1, 2, 2, 1, 2, 2, 2, 2, 2, 2, 2, 2, 1, 2, 2, 2, 2, 2, 2, 2, 2, 2, 1, 1, 1, 2, 2, 2, 1, 1, 2, 2, 1, 2, 4 ),
 ( 0.000000000000000000, 0.02254148184236093658, 0.03381222276354139966, 0.03944759322413162600, 0.04508296368472185234, 0.06762444552708282708, 0.07044213075737798535, 0.07114655206495175410, 0.07149876271873865929, 0.07185097337252556449, 0.07325981598767324077, 0.07889518644826387650, 0.09016592736944517572, 0.1127074092118077603, 0.1352488910541703448, 0.1408842615147609667, 0.1422931041299086152, 0.1429975254374824534, 0.1437019467450562915, 0.1465196319753516718, 0.1577903728965331376, 0.1803318547388961246, 0.1916025956600775904, 0.1944202808903729707, 0.1958291235055207025, 0.1961813341593076354, 0.1965335448130945684, 0.1972379661206684898, 0.2028733365812608325, 0.2254148184236299257, 0.2479563002659990467, 0.2493651428811471116, 0.2497173535349341555, 0.2500695641887212273, 0.2507739854962953152, 0.2535916707265916670, 0.2592270411871845370, 0.2704977821083701661, 0.2817685230295557952, 0.2845862082598522025, 0.2859950508750004339, 0.2874038934901486653, 0.2930392639507415908, 0.3155807457931132376, 0.3212161162537061077, 0.3213922215805997129, 0.3215683269074932626, 0.3219205375612803621, 0.3226249588688546166, 0.3240338014840031811, 0.3268514867143001990, 0.3381222276354884371, 0.3606637094778649688, 0.3832051913202414450, 0.3888405617808354808, 0.3916582470111326097, 0.3930670896262811187, 0.3944759322414296276, 0.4057466731626182543, 0.4282881550049952857, 0.4395588959261836903, 0.4451942663867780037, 0.4458986876943522581, 0.4466031090019265126, 0.4480119516170751881, 0.4508296368473724836, 0.4733711186897506251, 0.4959126005321287667, 0.4987302857624259511, 0.4994347070700003166, 0.5001391283775746821, 0.5015479709927231911, 0.5071833414533171158, 0.5184540823745051874, 0.5297248232956932590, 0.5353601937562872948, 0.5381778789865843127, 0.5409955642168814416, 0.5635370460592578068, 0.5691724165198518426, 0.5705812591350003515, 0.5712856804425746615, 0.5719901017501488605, 0.5748077869804457674, 0.5860785279016335059, 0.6086200097440088719, 0.6311614915863842379, 0.6424322325075718654, 0.6427844431613589649, 0.6431366538151460643, 0.6438410751227201523, 0.6452499177378684392, 0.6480676029681649020, 0.6537029734287579386, 0.6762444552711299739, 0.6875151961923159361, 0.6931505666529089726, 0.6959682518832054354, 0.6963204625369925349, 0.6966726731907795234, 0.6973770944983537223, 0.6987859371135020092, 0.7213274189558753768 ),
 .UNSPECIFIED. ) ;
#35250=CARTESIAN_POINT ( 'NONE',  ( -5.602526181104785508, -79.32510020630215308, 7.672075667186650350 ) ) ;
#35255=ORIENTED_EDGE ( 'NONE', *, *, #44519, .T. ) ;
#35280=DIRECTION ( 'NONE',  ( 0.000000000000000000, 1.000000000000000000, 0.000000000000000000 ) ) ;
#35283=CARTESIAN_POINT ( 'NONE',  ( 4.044903269867999640, -79.05999999999998806, -8.595856998426999240 ) ) ;
#35308=VERTEX_POINT ( 'NONE', #1652 ) ;
#35330=CARTESIAN_POINT ( 'NONE',  ( 0.000000000000000000, -75.20000000000000284, 0.000000000000000000 ) ) ;
#35333=CARTESIAN_POINT ( 'NONE',  ( -6.519655663280999214, -77.25306001420199209, 7.413858028194999505 ) ) ;
#35384=CARTESIAN_POINT ( 'NONE',  ( 0.000000000000000000, -75.20000000000000284, 7.200000000000000178 ) ) ;
#35408=CARTESIAN_POINT ( 'NONE',  ( -4.911790911253000047, -77.46226498579800079, -8.407543791226999019 ) ) ;
#35409=CARTESIAN_POINT ( 'NONE',  ( 6.055527902613000002, -77.71999999999999886, 7.319875806370000682 ) ) ;
#35422=CARTESIAN_POINT ( 'NONE',  ( -9.646692012709999986, -78.62005194988499568, 1.218660606027000215 ) ) ;
#35428=CARTESIAN_POINT ( 'NONE',  ( 5.365645860858371030, -78.12749999999998352, 7.890595865543487797 ) ) ;
#35455=ADVANCED_FACE ( 'NONE', ( #56246, #52109, #49349, #8896 ), #52397, .F. ) ;
#35457=CARTESIAN_POINT ( 'NONE',  ( 7.483407197968000801, -79.75000000000000000, -5.437013583705000208 ) ) ;
#35459=CONICAL_SURFACE ( 'NONE', #41265, 9.349999999968000353, 0.7853981633972997312 ) ;
#35462=CARTESIAN_POINT ( 'NONE',  ( -0.1199120982448000083, -77.75333998579800721, -9.541815775584998605 ) ) ;
#35478=CARTESIAN_POINT ( 'NONE',  ( -8.958921704583302059, -79.42676566002430150, -3.161023900737553127 ) ) ;
#35505=CARTESIAN_POINT ( 'NONE',  ( 11.65000000000000036, -75.20000000000000284, 0.000000000000000000 ) ) ;
#35510=CARTESIAN_POINT ( 'NONE',  ( 8.300970689365456678, -77.50833333333332575, -4.784380313523530326 ) ) ;
#35532=DIRECTION ( 'NONE',  ( 0.000000000000000000, 1.000000000000000000, 0.000000000000000000 ) ) ;
#35535=ORIENTED_EDGE ( 'NONE', *, *, #8970, .F. ) ;
#35540=VECTOR ( 'NONE', #26922, 1000.000000000000000 ) ;
#35548=CARTESIAN_POINT ( 'NONE',  ( -1.341561494378749719, -79.28604399664807545, 9.404764964287370077 ) ) ;
#35549=ORIENTED_EDGE ( 'NONE', *, *, #10925, .T. ) ;
#35566=CARTESIAN_POINT ( 'NONE',  ( 5.256696614975999715, -77.33533667140099510, 7.937185564810000038 ) ) ;
#35603=CARTESIAN_POINT ( 'NONE',  ( 0.000000000000000000, -77.00000000000000000, 0.000000000000000000 ) ) ;
#35611=EDGE_CURVE ( 'NONE', #4309, #13771, #4360, .T. ) ;
#35630=CARTESIAN_POINT ( 'NONE',  ( 4.993566916646000386, -77.65346001420199684, 8.516776984568000586 ) ) ;
#35656=DIRECTION ( 'NONE',  ( 1.000000000000000000, 0.000000000000000000, 0.000000000000000000 ) ) ;
#35658=CARTESIAN_POINT ( 'NONE',  ( 0.000000000000000000, -74.70999999999999375, 0.000000000000000000 ) ) ;
#35663=CARTESIAN_POINT ( 'NONE',  ( 0.000000000000000000, -74.70999999999999375, 0.000000000000000000 ) ) ;
#35666=CARTESIAN_POINT ( 'NONE',  ( 9.555317380607998956, -79.58626001420199714, 1.897550461403999966 ) ) ;
#35679=ORIENTED_EDGE ( 'NONE', *, *, #42096, .F. ) ;
#35692=CARTESIAN_POINT ( 'NONE',  ( -8.123853732960998997, -77.14685584965400267, 4.915330883505999893 ) ) ;
#35713=CARTESIAN_POINT ( 'NONE',  ( -2.715334531406999652, -77.04536332859899517, -9.237819267638000653 ) ) ;
#35725=ADVANCED_FACE ( 'NONE', ( #44250 ), #6715, .F. ) ;
#35727=CARTESIAN_POINT ( 'NONE',  ( 8.384816012895999648, -78.71759415034600238, -4.923277454554000343 ) ) ;
#35733=CARTESIAN_POINT ( 'NONE',  ( -6.954077596906954817, -78.23999999999998067, 6.533946999607151973 ) ) ;
#35761=CARTESIAN_POINT ( 'NONE',  ( 4.826563570534999847, -77.46213998579800375, 8.231944463396999367 ) ) ;
#35771=CARTESIAN_POINT ( 'NONE',  ( 0.000000000000000000, -74.70999999999999375, 0.000000000000000000 ) ) ;
#35780=CARTESIAN_POINT ( 'NONE',  ( -9.041368304669726186, -79.42452246446772790, -2.915530444129728949 ) ) ;
#35782=PLANE ( 'NONE',  #39350 ) ;
#35797=CARTESIAN_POINT ( 'NONE',  ( 9.500000000000000000, -78.54999999999999716, 0.000000000000000000 ) ) ;
#35809=CARTESIAN_POINT ( 'NONE',  ( 7.596835002782722057, -77.49791666666669698, -5.838193839761678383 ) ) ;
#35810=DIRECTION ( 'NONE',  ( 0.000000000000000000, 1.000000000000000000, 0.000000000000000000 ) ) ;
#35815=AXIS2_PLACEMENT_3D ( 'NONE', #35603, #5209, #18498 ) ;
#35826=CARTESIAN_POINT ( 'NONE',  ( 0.000000000000000000, -75.00000000000000000, -7.200000000000000178 ) ) ;
#35848=CARTESIAN_POINT ( 'NONE',  ( -3.621422511114219311, -79.30579764322290259, 8.782465238366681248 ) ) ;
#35860=ADVANCED_FACE ( 'NONE', ( #45637 ), #43912, .F. ) ;
#35885=CARTESIAN_POINT ( 'NONE',  ( 4.099012831087000208, -79.16778667140098946, -8.483720866318000375 ) ) ;
#35923=CARTESIAN_POINT ( 'NONE',  ( 9.209295719246959777, -79.54427083332929271, 2.475804444607904831 ) ) ;
#35929=AXIS2_PLACEMENT_3D ( 'NONE', #35384, #53411, #13257 ) ;
#35932=CARTESIAN_POINT ( 'NONE',  ( 7.661108911051000447, -77.95368667140100172, -6.051246682538999444 ) ) ;
#35940=CARTESIAN_POINT ( 'NONE',  ( -8.630067035710000667, -79.68530095943377489, -4.100810385846999750 ) ) ;
#35965=CARTESIAN_POINT ( 'NONE',  ( 9.500000000000000000, -78.06166666666669585, 1.392772743091435839 ) ) ;
#35967=FACE_OUTER_BOUND ( 'NONE', #27984, .T. ) ;
#35968=ORIENTED_EDGE ( 'NONE', *, *, #29217, .F. ) ;
#35990=CARTESIAN_POINT ( 'NONE',  ( -9.454379850511999805, -77.56257305011499170, 0.8787206290761000460 ) ) ;
#36001=CARTESIAN_POINT ( 'NONE',  ( -2.486604901413195456, -77.69583333333333997, 9.252740428348991131 ) ) ;
#36008=DIRECTION ( 'NONE',  ( -1.000000000000000000, 0.000000000000000000, 0.000000000000000000 ) ) ;
#36011=CARTESIAN_POINT ( 'NONE',  ( -8.944649069631999794, -77.41293832859899737, 3.564210769743999752 ) ) ;
#36023=CARTESIAN_POINT ( 'NONE',  ( 7.048436826466999428, -77.81756081701298911, 6.223291978577000449 ) ) ;
#36030=CARTESIAN_POINT ( 'NONE',  ( -0.6017968039497370025, -78.18000000000000682, 9.523103445003336276 ) ) ;
#36033=EDGE_CURVE ( 'NONE', #35308, #22854, #58056, .T. ) ;
#36035=B_SPLINE_CURVE_WITH_KNOTS ( 'NONE', 3,
 ( #33464, #42346, #47664, #50915, #34036, #24032 ),
 .UNSPECIFIED., .F., .F.,
 ( 4, 2, 4 ),
 ( 0.000000000000000000, 0.5000000000000000000, 1.000000000000000000 ),
 .UNSPECIFIED. ) ;
#36052=ADVANCED_FACE ( 'NONE', ( #51519 ), #11078, .T. ) ;
#36061=CARTESIAN_POINT ( 'NONE',  ( 4.959417147384999502, -77.95960665246400367, 7.893364288540000828 ) ) ;
#36069=CARTESIAN_POINT ( 'NONE',  ( 5.259675013629999896, -79.30162331913099649, -7.751687108632999035 ) ) ;
#36073=CARTESIAN_POINT ( 'NONE',  ( -2.364683833628040688, -79.44460282387935024, 9.258118656371037147 ) ) ;
#36078=CARTESIAN_POINT ( 'NONE',  ( 4.784380313523554307, -77.56666666666666288, -8.300970689365442468 ) ) ;
#36082=CARTESIAN_POINT ( 'NONE',  ( -5.397519881558073607, -79.47672766764729602, -7.818984972944852174 ) ) ;
#36113=AXIS2_PLACEMENT_3D ( 'NONE', #53750, #21852, #9169 ) ;
#36150=CARTESIAN_POINT ( 'NONE',  ( -9.473686928965467047, -79.39394681044888102, 0.7053954857237642040 ) ) ;
#36210=ORIENTED_EDGE ( 'NONE', *, *, #24530, .F. ) ;
#36269=CARTESIAN_POINT ( 'NONE',  ( 8.346732565571000961, -79.46528667140100310, -4.809657925418000524 ) ) ;
#36290=CARTESIAN_POINT ( 'NONE',  ( -9.454379850511999805, -77.62267694988499045, 0.8787206290761000460 ) ) ;
#36307=CARTESIAN_POINT ( 'NONE',  ( -4.857034759904000687, -77.52603832859900024, -8.313817338163000059 ) ) ;
#36320=CARTESIAN_POINT ( 'NONE',  ( -3.339615680726000235, -78.41274415034598633, 9.131854552393999569 ) ) ;
#36351=CARTESIAN_POINT ( 'NONE',  ( 4.784380313523554307, -78.56666666666666288, -8.300970689365442468 ) ) ;
#36359=CARTESIAN_POINT ( 'NONE',  ( -5.580112777935000601, -78.05318998579799938, 7.918523194479999638 ) ) ;
#36362=CARTESIAN_POINT ( 'NONE',  ( 5.645589344077617255, -79.37440282387937884, 7.709202350186582287 ) ) ;
#36396=CARTESIAN_POINT ( 'NONE',  ( 8.256620083228000340, -77.35889903538301837, -4.688888258373000717 ) ) ;
#36401=CARTESIAN_POINT ( 'NONE',  ( -1.243547092045951041, -77.41458333333332575, -9.500000000000000000 ) ) ;
#36455=CARTESIAN_POINT ( 'NONE',  ( 5.320338141332999982, -79.17917000473400435, -7.841092173349999861 ) ) ;
#36472=CARTESIAN_POINT ( 'NONE',  ( -9.519228660049000368, -79.57086001420199750, -0.02392464561790000332 ) ) ;
#36499=VERTEX_POINT ( 'NONE', #55132 ) ;
#36513=DIRECTION ( 'NONE',  ( -3.497202527557000183E-12, 1.000000000000000000, -1.787423860910000090E-11 ) ) ;
#36518=CARTESIAN_POINT ( 'NONE',  ( 4.242467933327000118, -77.84428667140100799, 8.300509423296000833 ) ) ;
#36525=CARTESIAN_POINT ( 'NONE',  ( -4.371390937481000272, -77.78071332859899201, -8.606055931584998930 ) ) ;
#36561=CARTESIAN_POINT ( 'NONE',  ( -9.392797912344001077, -79.62373998579799661, 0.6620803225204999753 ) ) ;
#36565=CARTESIAN_POINT ( 'NONE',  ( -9.312500000004000356, -79.68749999999599254, 6.570867420027000168E-10 ) ) ;
#36571=LINE ( 'NONE', #46333, #26370 ) ;
#36580=CARTESIAN_POINT ( 'NONE',  ( -4.802567994450000377, -77.15274805011500803, -8.191018798270000900 ) ) ;
#36598=CARTESIAN_POINT ( 'NONE',  ( 7.864930754364000798, -77.17951498579800784, 5.740674767402000001 ) ) ;
#36625=CARTESIAN_POINT ( 'NONE',  ( 9.500000000000000000, -79.14999999999999147, 0.000000000000000000 ) ) ;
#36653=CARTESIAN_POINT ( 'NONE',  ( 9.540055299840034309, -79.30420282387936481, 0.5400507987868797821 ) ) ;
#36688=CARTESIAN_POINT ( 'NONE',  ( 9.475051992780000987, -77.89482403538302435, -0.6170397550469999270 ) ) ;
#36694=CARTESIAN_POINT ( 'NONE',  ( 0.7264933893478244809, -79.75000000000000000, -9.249999992442631935 ) ) ;
#36707=VECTOR ( 'NONE', #52743, 1000.000000000000114 ) ;
#36725=CARTESIAN_POINT ( 'NONE',  ( 5.441664396738000065, -79.49294334753599856, -8.019902302782998760 ) ) ;
#36731=FACE_OUTER_BOUND ( 'NONE', #395, .T. ) ;
#36739=CARTESIAN_POINT ( 'NONE',  ( -2.664101853300902434, -77.15209693750341557, -9.063520957256455901 ) ) ;
#36740=CARTESIAN_POINT ( 'NONE',  ( 0.000000000000000000, -75.00000000000000000, -7.200000000000000178 ) ) ;
#36745=CARTESIAN_POINT ( 'NONE',  ( -8.885605805125999623, -78.03806001420198868, 3.858414063430999796 ) ) ;
#36774=ORIENTED_EDGE ( 'NONE', *, *, #3067, .T. ) ;
#36786=B_SPLINE_SURFACE_WITH_KNOTS ( 'NONE', 3, 3, ( 
 ( #25051, #43073, #34470, #56647, #34181, #52501, #12059, #20628, #40065, #3482, #53961, #44805, #40371, #58082, #44503, #35630, #48940, #58379, #17641, #17060, #31193, #17941, #4661, #22661, #49536, #25911, #35333, #35041, #18244, #53075, #30622, #30329, #27069, #12626, #26775 ),
 ( #45108, #48655, #31490, #52787, #9083, #35932, #13498, #8199, #53658, #48371, #53359, #40671, #261, #12342, #49232, #26201, #21487, #3768, #7909, #12907, #44219, #30905, #43933, #39494, #57498, #21771, #4356, #39774, #57789, #17344, #22358, #8485, #26480, #4054, #22058 ),
 ( #13198, #8784, #14960, #23819, #32957, #27658, #5814, #18533, #36525, #37103, #51002, #32087, #41838, #10551, #41252, #28533, #24116, #5521, #23244, #1700, #13789, #9380, #50127, #45701, #5239, #839, #18822, #36814, #54832, #32373, #57624, #17472, #27189, #40199, #49660 ),
 ( #8323, #36061, #44337, #49067, #39901, #57915, #45229, #35462, #13620, #53791, #13031, #26903, #8913, #40496, #4191, #35761, #44931, #39333, #4488, #22486, #93, #42767, #51634, #42181, #10897, #11476, #11188, #27485, #29164, #47211, #6446, #51916, #1750, #38318, #45526 ) ),
 .UNSPECIFIED., .F., .F., .F.,
 ( 4, 4 ),
 ( 4, 1, 1, 1, 1, 1, 1, 1, 1, 1, 1, 1, 1, 1, 1, 1, 1, 1, 1, 1, 1, 1, 1, 1, 1, 1, 1, 1, 1, 1, 1, 1, 4 ),
 ( -0.1377334280162000046, 1.137733428016000081 ),
 ( -0.01671641791045000089, 0.01044776119403000025, 0.03761194029850999793, 0.06477611940298999560, 0.09194029850746000820, 0.1191044776118999893, 0.1462686567163999918, 0.1734328358208999943, 0.2005970149253999968, 0.2277611940298999993, 0.2549253731343000262, 0.2820895522388000010, 0.3092537313432999757, 0.3364179104478000060, 0.3635820895522000051, 0.3907462686567000354, 0.4179104477612000101, 0.4450746268656999849, 0.4722388059701999596, 0.4994029850746000143, 0.5265671641790999891, 0.5537313432836000748, 0.5808955223881000496, 0.6080597014924999932, 0.6352238805969999680, 0.6623880597014999427, 0.6895522388060000285, 0.7167164179105000033, 0.7438805970148999469, 0.7710447761194000327, 0.7982089552239000074, 0.8253731343283999822, 0.8525373134328000368 ),
 .UNSPECIFIED. ) ;
#36794=ORIENTED_EDGE ( 'NONE', *, *, #16973, .F. ) ;
#36814=CARTESIAN_POINT ( 'NONE',  ( -2.517806253849999898, -77.08911332859899801, 9.318471479766001764 ) ) ;
#36849=CARTESIAN_POINT ( 'NONE',  ( 0.000000000000000000, -79.79999999999999716, 0.000000000000000000 ) ) ;
#36868=CARTESIAN_POINT ( 'NONE',  ( 2.962511214703000384, -77.78030194988500057, -9.021140561863999707 ) ) ;
#36878=CARTESIAN_POINT ( 'NONE',  ( -9.500000000000000000, -77.79999999999999716, 0.000000000000000000 ) ) ;
#36895=CARTESIAN_POINT ( 'NONE',  ( 7.377665174502719303, -77.00000000000001421, 5.715929696616472100 ) ) ;
#36922=CARTESIAN_POINT ( 'NONE',  ( -7.934077584064515243, -77.00000000000000000, -5.060727184842107818 ) ) ;
#36927=CARTESIAN_POINT ( 'NONE',  ( -4.658152026654871491, -79.73958333333277437, -8.062158950714737315 ) ) ;
#36931=CARTESIAN_POINT ( 'NONE',  ( 7.184181682494999777, -77.75082999526600247, 6.343145485738000744 ) ) ;
#36950=LINE ( 'NONE', #1258, #32860 ) ;
#36956=CARTESIAN_POINT ( 'NONE',  ( 4.044903269867999640, -79.46000000000000796, -8.595856998426999240 ) ) ;
#36978=CARTESIAN_POINT ( 'NONE',  ( 4.574312611392000072, -77.48499903538302647, 8.320643751074999983 ) ) ;
#36984=CARTESIAN_POINT ( 'NONE',  ( 1.000000000000000000, -78.00000000000000000, 7.200000000000000178 ) ) ;
#36997=CARTESIAN_POINT ( 'NONE',  ( -5.838193839761688153, -77.87291666666668277, -7.596835002782716728 ) ) ;
#37017=CARTESIAN_POINT ( 'NONE',  ( -9.896988620242000323, -79.33326001420199702, -1.580285165976000217 ) ) ;
#37031=ADVANCED_FACE ( 'NONE', ( #53986 ), #30355, .T. ) ;
#37040=DIRECTION ( 'NONE',  ( 0.000000000000000000, -1.000000000000000000, 0.000000000000000000 ) ) ;
#37069=DIRECTION ( 'NONE',  ( 1.000000000000000000, 0.000000000000000000, 0.000000000000000000 ) ) ;
#37098=CARTESIAN_POINT ( 'NONE',  ( 9.027899509543001244, -77.73118667140099092, -3.021393903538999837 ) ) ;
#37103=CARTESIAN_POINT ( 'NONE',  ( -7.722699735758999928, -77.74431332859899157, -5.790782847811000167 ) ) ;
#37162=CARTESIAN_POINT ( 'NONE',  ( -2.205007487985999770, -77.02370194988500884, 9.235565851336001941 ) ) ;
#37213=CARTESIAN_POINT ( 'NONE',  ( -3.655354238636269848, -77.00000000000000000, -8.765527374921106230 ) ) ;
#37218=CARTESIAN_POINT ( 'NONE',  ( -9.147655554837982095, -79.69791666666337449, -1.948585094003928431 ) ) ;
#37221=CARTESIAN_POINT ( 'NONE',  ( -5.674993058560000136, -78.45643998579799927, -8.260872093916999503 ) ) ;
#37236=VERTEX_POINT ( 'NONE', #24140 ) ;
#37268=CYLINDRICAL_SURFACE ( 'NONE', #29539, 1.000000000000000000 ) ;
#37306=CARTESIAN_POINT ( 'NONE',  ( 6.874531804813999614, -78.50581001420199811, -7.293035489291000317 ) ) ;
#37346=CARTESIAN_POINT ( 'NONE',  ( -2.437266298365000416, -79.27423998579799047, 9.542290714110000849 ) ) ;
#37355=CARTESIAN_POINT ( 'NONE',  ( -6.053394164830000257, -79.70045194988499304, -7.392643757108000813 ) ) ;
#37359=CARTESIAN_POINT ( 'NONE',  ( -9.199999999999999289, -80.59999999999999432, 0.000000000000000000 ) ) ;
#37364=LINE ( 'NONE', #19372, #5813 ) ;
#37370=AXIS2_PLACEMENT_3D ( 'NONE', #56587, #56881, #57158 ) ;
#37374=CARTESIAN_POINT ( 'NONE',  ( 9.499988113994666250, -79.15199854361453902, 0.2409522322386896676 ) ) ;
#37389=CARTESIAN_POINT ( 'NONE',  ( 6.619314962793000134, -77.25773501420199807, -6.690398925867999225 ) ) ;
#37405=CARTESIAN_POINT ( 'NONE',  ( -9.646692012709999986, -78.49984415034599294, 1.218660606027000215 ) ) ;
#37444=DIRECTION ( 'NONE',  ( 0.000000000000000000, 0.7071067811866525998, -0.7071067811864425456 ) ) ;
#37448=DIRECTION ( 'NONE',  ( 0.000000000000000000, -1.000000000000000000, 0.000000000000000000 ) ) ;
#37449=ORIENTED_EDGE ( 'NONE', *, *, #37684, .F. ) ;
#37452=CARTESIAN_POINT ( 'NONE',  ( -9.061228178001998756, -77.53399415034598974, -2.837532765875999896 ) ) ;
#37467=B_SPLINE_CURVE_WITH_KNOTS ( 'NONE', 3,
 ( #29084, #50960, #56257, #15219, #10216, #15516, #55669, #28789, #10511, #47129 ),
 .UNSPECIFIED., .F., .F.,
 ( 4, 2, 2, 2, 4 ),
 ( 0.000000000000000000, 0.1874999983493903788, 0.3749999966987807576, 0.5624999950481708311, 0.7499999933975610711 ),
 .UNSPECIFIED. ) ;
#37501=EDGE_CURVE ( 'NONE', #89, #14353, #28582, .T. ) ;
#37512=VERTEX_POINT ( 'NONE', #58339 ) ;
#37600=CARTESIAN_POINT ( 'NONE',  ( 2.278690965393999956, -79.46391001420199984, -9.759650287631000509 ) ) ;
#37615=CARTESIAN_POINT ( 'NONE',  ( -5.650756493884554033, -77.12382193750340775, -7.570587593239054947 ) ) ;
#37626=CARTESIAN_POINT ( 'NONE',  ( 3.938458446976999205, -79.21000000000000796, -8.369650235310999165 ) ) ;
#37640=CARTESIAN_POINT ( 'NONE',  ( -9.848602347018999836, -79.37953998579800441, -0.02475245940598000058 ) ) ;
#37646=CARTESIAN_POINT ( 'NONE',  ( -7.530775182571000315, -78.20449514476064223, -6.150709233331998149 ) ) ;
#37651=CARTESIAN_POINT ( 'NONE',  ( 1.813979036992999783, -79.54995584965399757, 9.381055131006998948 ) ) ;
#37668=CARTESIAN_POINT ( 'NONE',  ( 4.060630270881947723, -79.23944037031237997, 8.588476052470577216 ) ) ;
#37684=EDGE_CURVE ( 'NONE', #5875, #31891, #7697, .T. ) ;
#37723=VERTEX_POINT ( 'NONE', #19945 ) ;
#37739=ADVANCED_FACE ( 'NONE', ( #37934 ), #52199, .F. ) ;
#37759=AXIS2_PLACEMENT_3D ( 'NONE', #44923, #23357, #373 ) ;
#37800=CARTESIAN_POINT ( 'NONE',  ( -8.764769494928954074, -76.99999999999998579, -3.351978445651452532 ) ) ;
#37806=CARTESIAN_POINT ( 'NONE',  ( -2.858407197967999913, -79.75000000000000000, -8.797272775729998884 ) ) ;
#37809=CARTESIAN_POINT ( 'NONE',  ( 9.665471083832999355, -78.10803998579800123, -2.650702293911000318 ) ) ;
#37835=B_SPLINE_CURVE_WITH_KNOTS ( 'NONE', 3,
 ( #31618, #49659, #45228, #17471, #13030, #49066, #36351, #40494, #31319, #3606, #4776, #9204, #4190, #49363, #31910, #27188, #48779, #40785 ),
 .UNSPECIFIED., .F., .F.,
 ( 4, 2, 2, 2, 2, 2, 2, 2, 4 ),
 ( 0.000000000000000000, 0.1249999999999999445, 0.2499999999999998890, 0.3749999999999998335, 0.4999999999999997780, 0.6249999999999997780, 0.7499999999999997780, 0.8749999999999997780, 1.000000000000000000 ),
 .UNSPECIFIED. ) ;
#37838=ORIENTED_EDGE ( 'NONE', *, *, #15455, .T. ) ;
#37848=CARTESIAN_POINT ( 'NONE',  ( 4.316051676898999823, -79.02855584965399771, 8.712949996777000550 ) ) ;
#37865=ORIENTED_EDGE ( 'NONE', *, *, #44501, .F. ) ;
#37868=B_SPLINE_CURVE_WITH_KNOTS ( 'NONE', 3,
 ( #19406, #5524, #14376, #45111, #41841, #55122, #45703, #32376, #14963, #32663, #31792, #50716, #10257, #27949, #32960, #23246, #1416, #49835 ),
 .UNSPECIFIED., .F., .F.,
 ( 4, 2, 2, 2, 2, 2, 2, 2, 4 ),
 ( 0.000000000000000000, 0.1250000000000000555, 0.2500000000000001110, 0.3750000000000001665, 0.5000000000000002220, 0.6250000000000001110, 0.7500000000000001110, 0.8750000000000000000, 1.000000000000000000 ),
 .UNSPECIFIED. ) ;
#37910=CARTESIAN_POINT ( 'NONE',  ( 4.399173910654000430, -78.78151332859899014, 8.880751478442000746 ) ) ;
#37917=DIRECTION ( 'NONE',  ( 0.000000000000000000, 0.000000000000000000, -1.000000000000000000 ) ) ;
#37929=CARTESIAN_POINT ( 'NONE',  ( 6.603857951666999959, -79.12741332859900467, -7.157719488480999814 ) ) ;
#37934=FACE_OUTER_BOUND ( 'NONE', #50744, .T. ) ;
#37952=EDGE_LOOP ( 'NONE', ( #25367, #22780, #17100, #2547, #56843 ) ) ;
#37957=CARTESIAN_POINT ( 'NONE',  ( 7.172098529503864839, -79.20654853075065205, 6.236001066935767945 ) ) ;
#37972=CARTESIAN_POINT ( 'NONE',  ( -5.148784662568076406E-06, -79.56241750339395935, -9.437165819784945953 ) ) ;
#38039=CARTESIAN_POINT ( 'NONE',  ( -5.597970637881999778, -76.93501915034599392, 7.669424558767000022 ) ) ;
#38043=CARTESIAN_POINT ( 'NONE',  ( 6.585541864823201585, -78.36492913613842859, 7.155704809941277666 ) ) ;
#38081=ORIENTED_EDGE ( 'NONE', *, *, #24108, .F. ) ;
#38099=ORIENTED_EDGE ( 'NONE', *, *, #15132, .T. ) ;
#38100=CARTESIAN_POINT ( 'NONE',  ( -6.954077596906954817, -77.83999999999998920, 6.533946999607151085 ) ) ;
#38102=EDGE_LOOP ( 'NONE', ( #30151, #14055, #52064, #29228 ) ) ;
#38104=CARTESIAN_POINT ( 'NONE',  ( -9.452993584203847277, -79.39181711029749522, 0.9501152051606440718 ) ) ;
#38134=CARTESIAN_POINT ( 'NONE',  ( -0.5312504855272001114, -78.81080584965400249, -9.708839960653000034 ) ) ;
#38183=CARTESIAN_POINT ( 'NONE',  ( -0.5353773281849999455, -78.81376332859899492, -9.784259853904000437 ) ) ;
#38202=CARTESIAN_POINT ( 'NONE',  ( -8.988089064694998243, -77.97428667140098923, 3.902915570549000179 ) ) ;
#38207=CYLINDRICAL_SURFACE ( 'NONE', #1584, 9.199999999999999289 ) ;
#38232=CARTESIAN_POINT ( 'NONE',  ( -2.364557222828000072, -79.52495194988499350, 9.257622954664000758 ) ) ;
#38236=CARTESIAN_POINT ( 'NONE',  ( 9.500000000000001776, -77.16041666666667709, 1.243547092045981239 ) ) ;
#38238=DIRECTION ( 'NONE',  ( 0.000000000000000000, 1.000000000000000000, 0.000000000000000000 ) ) ;
#38248=CARTESIAN_POINT ( 'NONE',  ( 2.135299940751924197, -79.25691378410574828, 9.265864175146425907 ) ) ;
#38316=ORIENTED_EDGE ( 'NONE', *, *, #41867, .F. ) ;
#38318=CARTESIAN_POINT ( 'NONE',  ( 6.766607812238000008, -76.81907331913100734, -6.412022843746999712 ) ) ;
#38325=FACE_OUTER_BOUND ( 'NONE', #20766, .T. ) ;
#38336=CARTESIAN_POINT ( 'NONE',  ( 4.784380313523554307, -78.06666666666666288, -8.300970689365442468 ) ) ;
#38340=CARTESIAN_POINT ( 'NONE',  ( 1.243547092045927949, -78.76458333333332007, 9.500000000000003553 ) ) ;
#38346=EDGE_LOOP ( 'NONE', ( #6373, #20046 ) ) ;
#38396=FACE_OUTER_BOUND ( 'NONE', #7755, .T. ) ;
#38409=CARTESIAN_POINT ( 'NONE',  ( -9.199999999999999289, -76.00000000000000000, 0.000000000000000000 ) ) ;
#38435=DIRECTION ( 'NONE',  ( 1.000000000000000000, 0.000000000000000000, 0.000000000000000000 ) ) ;
#38444=CARTESIAN_POINT ( 'NONE',  ( 0.000000000000000000, -75.00000000000000000, 7.200000000000000178 ) ) ;
#38457=PRODUCT ( 'Push Button Cover', 'Push Button Cover', '', ( #55615 ) ) ;
#38474=CARTESIAN_POINT ( 'NONE',  ( 8.283364115789000337, -78.98796332859900815, 5.234906771447999319 ) ) ;
#38485=CARTESIAN_POINT ( 'NONE',  ( -9.400098536042321484, -79.41121447921612742, -1.373460959377882817 ) ) ;
#38493=CARTESIAN_POINT ( 'NONE',  ( 1.914689014128999833, -78.36623667140099769, 9.610012265935001352 ) ) ;
#38514=CARTESIAN_POINT ( 'NONE',  ( 6.954077596906981462, -79.08999999999998920, -6.533946999607122663 ) ) ;
#38521=CARTESIAN_POINT ( 'NONE',  ( -7.603664017117999663, -78.59644514476066490, 6.060370778711000384 ) ) ;
#38524=CARTESIAN_POINT ( 'NONE',  ( 1.813979036992999783, -79.36964415034600506, 9.381055131006998948 ) ) ;
#38531=CARTESIAN_POINT ( 'NONE',  ( 5.838193839761673054, -78.62291666666669698, 7.596835002782728274 ) ) ;
#38540=CARTESIAN_POINT ( 'NONE',  ( 6.480685897343804847, -79.21501409628969270, 6.948370975495136825 ) ) ;
#38542=ORIENTED_EDGE ( 'NONE', *, *, #44273, .T. ) ;
#38547=CARTESIAN_POINT ( 'NONE',  ( -2.318113117698174186, -79.65520282387936390, -9.269879263659483115 ) ) ;
#38592=LINE ( 'NONE', #43321, #23596 ) ;
#38617=CARTESIAN_POINT ( 'NONE',  ( -9.391369684923001060, -76.99806915034599797, 1.399863080762999923 ) ) ;
#38629=CARTESIAN_POINT ( 'NONE',  ( -9.500000000000001776, -77.91041666666669130, -1.243547092045959923 ) ) ;
#38632=CARTESIAN_POINT ( 'NONE',  ( 0.000000000000000000, -80.59999999999999432, 0.000000000000000000 ) ) ;
#38637=ORIENTED_EDGE ( 'NONE', *, *, #43247, .F. ) ;
#38717=CARTESIAN_POINT ( 'NONE',  ( 9.377128579935000374, -78.35875194988499004, -2.571625947824999869 ) ) ;
#38724=CARTESIAN_POINT ( 'NONE',  ( 9.500000000000000000, -77.14999999999999147, 0.000000000000000000 ) ) ;
#38750=( LENGTH_UNIT ( ) NAMED_UNIT ( * ) SI_UNIT ( .MILLI., .METRE. ) );
#38762=CARTESIAN_POINT ( 'NONE',  ( -0.8644569908188000085, -79.13883667140099476, 9.872851397518997985 ) ) ;
#38779=CARTESIAN_POINT ( 'NONE',  ( -0.6596342590195000133, -77.82341332859900263, 9.888746480308999054 ) ) ;
#38807=B_SPLINE_CURVE_WITH_KNOTS ( 'NONE', 3,
 ( #14837, #36694, #50006, #9552, #10424, #23121, #45872, #5406, #1007, #18992 ),
 .UNSPECIFIED., .F., .F.,
 ( 4, 2, 2, 2, 4 ),
 ( 0.2500000082780876598, 0.4375000062085657726, 0.6250000041390437744, 0.8125000020695218872, 1.000000000000000000 ),
 .UNSPECIFIED. ) ;
#38830=CARTESIAN_POINT ( 'NONE',  ( 3.266878030750679951, -79.24670026210782225, 8.921992862818912684 ) ) ;
#38833=CARTESIAN_POINT ( 'NONE',  ( 0.000000000000000000, -79.65000000003199432, 0.000000000000000000 ) ) ;
#38859=CARTESIAN_POINT ( 'NONE',  ( -1.243547092045993674, -78.28541666666666288, 9.499999999999996447 ) ) ;
#38888=ORIENTED_EDGE ( 'NONE', *, *, #52146, .F. ) ;
#38906=CARTESIAN_POINT ( 'NONE',  ( 8.220803302871821927, -78.84397913613844366, 5.195369692238999804 ) ) ;
#38948=CARTESIAN_POINT ( 'NONE',  ( -3.046227980494999876, -79.91992668086899698, -9.106622846827001183 ) ) ;
#38956=CARTESIAN_POINT ( 'NONE',  ( -7.483407197968000801, -77.00000000000000000, 5.437013583706000297 ) ) ;
#38963=ORIENTED_EDGE ( 'NONE', *, *, #28974, .T. ) ;
#39008=CARTESIAN_POINT ( 'NONE',  ( -8.918806285220000518, -78.09745194988499861, 3.872830773119999570 ) ) ;
#39014=CARTESIAN_POINT ( 'NONE',  ( 0.000000000000000000, -75.20000000000000284, -8.199999999999999289 ) ) ;
#39048=CARTESIAN_POINT ( 'NONE',  ( -3.292576784871000140, -78.35493667140100627, -9.347695904456999827 ) ) ;
#39063=AXIS2_PLACEMENT_3D ( 'NONE', #45456, #54309, #24169 ) ;
#39069=CARTESIAN_POINT ( 'NONE',  ( -5.644471715163000169, -77.93073667140099303, 8.009852484315999277 ) ) ;
#39076=CARTESIAN_POINT ( 'NONE',  ( -7.596835002782709623, -78.85208333333333997, -5.838193839761696147 ) ) ;
#39099=EDGE_CURVE ( 'NONE', #21408, #11254, #37467, .T. ) ;
#39111=DIRECTION ( 'NONE',  ( 0.000000000000000000, 1.000000000000000000, 0.000000000000000000 ) ) ;
#39122=CARTESIAN_POINT ( 'NONE',  ( -6.579782092783524661, -79.33575076626789269, 6.852906106304269329 ) ) ;
#39140=CARTESIAN_POINT ( 'NONE',  ( 0.000000000000000000, -74.70999999999999375, 0.000000000000000000 ) ) ;
#39148=EDGE_CURVE ( 'NONE', #35206, #39734, #11463, .T. ) ;
#39213=AXIS2_PLACEMENT_3D ( 'NONE', #9686, #22970, #40980 ) ;
#39235=CARTESIAN_POINT ( 'NONE',  ( -9.337827476838000962, -79.84366001420200121, -2.776632127938000405 ) ) ;
#39245=VERTEX_POINT ( 'NONE', #37359 ) ;
#39252=CARTESIAN_POINT ( 'NONE',  ( -6.013262726775999489, -77.61973084965400460, 7.348341287529000176 ) ) ;
#39282=CARTESIAN_POINT ( 'NONE',  ( -6.173435753739000553, -76.93948667140098507, 6.984674784554999682 ) ) ;
#39294=CARTESIAN_POINT ( 'NONE',  ( -5.505695391233000002, -78.76725584965399207, -8.014431902511001127 ) ) ;
#39314=CIRCLE ( 'NONE', #26111, 11.44999999999999929 ) ;
#39318=CIRCLE ( 'NONE', #24232, 11.65000000000000036 ) ;
#39323=VECTOR ( 'NONE', #35810, 1000.000000000000000 ) ;
#39333=CARTESIAN_POINT ( 'NONE',  ( 9.467323119481999782, -77.38933998579800289, 1.196001045232000015 ) ) ;
#39342=CARTESIAN_POINT ( 'NONE',  ( 8.449950666592000559, -78.90086332859900153, -4.961522297560000183 ) ) ;
#39350=AXIS2_PLACEMENT_3D ( 'NONE', #4801, #49387, #9813 ) ;
#39395=CARTESIAN_POINT ( 'NONE',  ( 6.479078291783999966, -79.25424805011499529, -7.022474634662000170 ) ) ;
#39413=AXIS2_PLACEMENT_3D ( 'NONE', #58050, #17031, #52471 ) ;
#39416=CARTESIAN_POINT ( 'NONE',  ( -1.025492391311069618, -79.28331459140689219, 9.446644090482800848 ) ) ;
#39443=CARTESIAN_POINT ( 'NONE',  ( 5.838193839761669501, -78.22291666666666288, 7.596835002782726498 ) ) ;
#39463=CARTESIAN_POINT ( 'NONE',  ( 9.500000000000000000, -77.04999999999999716, 0.000000000000000000 ) ) ;
#39488=CARTESIAN_POINT ( 'NONE',  ( -5.751575620263249533, -79.64192708332932114, 7.482738016046601714 ) ) ;
#39494=CARTESIAN_POINT ( 'NONE',  ( -8.458823954585000138, -77.29848667140100815, -4.874260255650000317 ) ) ;
#39526=CARTESIAN_POINT ( 'NONE',  ( -7.678106106111999729, -79.80848667140099906, -5.817855318239999463 ) ) ;
#39535=DIRECTION ( 'NONE',  ( 1.000000000000000000, 0.000000000000000000, 0.000000000000000000 ) ) ;
#39545=B_SPLINE_CURVE_WITH_KNOTS ( 'NONE', 3,
 ( #14856, #6300, #32851, #15153 ),
 .UNSPECIFIED., .F., .F.,
 ( 4, 4 ),
 ( 0.000000000000000000, 1.000000000000000000 ),
 .UNSPECIFIED. ) ;
#39546=CARTESIAN_POINT ( 'NONE',  ( -1.269916711065999904, -77.30448084965399858, -9.409822520238998678 ) ) ;
#39580=LINE ( 'NONE', #48179, #14612 ) ;
#39583=CARTESIAN_POINT ( 'NONE',  ( -0.8481231068849000021, -79.01200194988500414, 9.686304223355000076 ) ) ;
#39598=DIRECTION ( 'NONE',  ( 0.000000000000000000, 1.000000000000000000, 0.000000000000000000 ) ) ;
#39606=CYLINDRICAL_SURFACE ( 'NONE', #33155, 5.100000000000000533 ) ;
#39623=CARTESIAN_POINT ( 'NONE',  ( -7.575359187103000380, -78.57578998579799645, 6.037810896484000267 ) ) ;
#39635=CARTESIAN_POINT ( 'NONE',  ( -3.989559569275991979, -79.49016193574067302, -8.633000817857986675 ) ) ;
#39640=CARTESIAN_POINT ( 'NONE',  ( -9.499653450934914645, -79.30027302004205580, 1.387647615217423080E-06 ) ) ;
#39648=CIRCLE ( 'NONE', #30246, 5.100000000000000533 ) ;
#39651=CARTESIAN_POINT ( 'NONE',  ( -4.784380313523538319, -78.88333333333333997, -8.300970689365453126 ) ) ;
#39657=ORIENTED_EDGE ( 'NONE', *, *, #53660, .T. ) ;
#39697=CARTESIAN_POINT ( 'NONE',  ( 1.449316606189569034, -79.26277057543936166, 9.388788162982219632 ) ) ;
#39714=CARTESIAN_POINT ( 'NONE',  ( 3.923097297260000005, -77.16568667140100501, -8.674161723994000539 ) ) ;
#39734=VERTEX_POINT ( 'NONE', #40905 ) ;
#39774=CARTESIAN_POINT ( 'NONE',  ( -2.546514579946999923, -77.15288667140099221, 9.424721798891001256 ) ) ;
#39820=VECTOR ( 'NONE', #32834, 1000.000000000000000 ) ;
#39823=ORIENTED_EDGE ( 'NONE', *, *, #19172, .T. ) ;
#39830=CARTESIAN_POINT ( 'NONE',  ( 5.807838419657000095, -77.36753084965400262, -7.511754867730999763 ) ) ;
#39852=CARTESIAN_POINT ( 'NONE',  ( 1.741786704463999857, -77.58258832859900167, -9.469768965712999531 ) ) ;
#39867=CARTESIAN_POINT ( 'NONE',  ( -3.039602602086000083, -79.22975194988498515, -9.236151215514999180 ) ) ;
#39883=DIRECTION ( 'NONE',  ( -1.000000000000000000, 0.000000000000000000, 0.000000000000000000 ) ) ;
#39884=ORIENTED_EDGE ( 'NONE', *, *, #16238, .F. ) ;
#39901=CARTESIAN_POINT ( 'NONE',  ( 9.330693044838000105, -77.86253998579799429, -1.999643576009999757 ) ) ;
#39909=CARTESIAN_POINT ( 'NONE',  ( -3.028287605162000240, -79.22903998579799634, -9.201769410957998829 ) ) ;
#39917=CARTESIAN_POINT ( 'NONE',  ( -5.838193839761687265, -77.47291666666666288, -7.596835002782715840 ) ) ;
#39956=DIRECTION ( 'NONE',  ( -1.000000000000000000, 0.000000000000000000, 0.000000000000000000 ) ) ;
#39975=EDGE_LOOP ( 'NONE', ( #13650, #13403, #29605, #31103, #29006, #29796, #19464, #39823 ) ) ;
#39986=CARTESIAN_POINT ( 'NONE',  ( -7.601074271102891800, -79.34838228251635428, 5.698502993689569252 ) ) ;
#40007=DIRECTION ( 'NONE',  ( 0.000000000000000000, 1.000000000000000000, 0.000000000000000000 ) ) ;
#40019=CARTESIAN_POINT ( 'NONE',  ( -6.067803813374999855, -79.50066001420199768, 7.334714833394000877 ) ) ;
#40025=EDGE_CURVE ( 'NONE', #1317, #10320, #54005, .T. ) ;
#40065=CARTESIAN_POINT ( 'NONE',  ( -4.471077175322999864, -77.90826001420199987, -8.802310476361999036 ) ) ;
#40073=CARTESIAN_POINT ( 'NONE',  ( -2.858407197967999913, -79.75000000000000000, -8.797272775729998884 ) ) ;
#40124=CARTESIAN_POINT ( 'NONE',  ( -9.204193785523999694, -77.20990584965399250, -2.332437886131999871 ) ) ;
#40129=EDGE_CURVE ( 'NONE', #10450, #31238, #14175, .T. ) ;
#40147=CARTESIAN_POINT ( 'NONE',  ( 9.233773875527001351, -77.60363998579799727, -3.090294488178999988 ) ) ;
#40160=CARTESIAN_POINT ( 'NONE',  ( 6.482950081930999531, -79.19664415034600324, -6.598019266050999754 ) ) ;
#40165=ORIENTED_EDGE ( 'NONE', *, *, #3067, .F. ) ;
#40166=CARTESIAN_POINT ( 'NONE',  ( -8.500869906239364227, -78.26250000000001705, 4.334382246026820873 ) ) ;
#40199=CARTESIAN_POINT ( 'NONE',  ( 6.844651340168000253, -76.88284666193300154, -6.485976721047999938 ) ) ;
#40207=CARTESIAN_POINT ( 'NONE',  ( -8.885605805125999623, -78.09673998579799559, 3.858414063430999796 ) ) ;
#40218=CARTESIAN_POINT ( 'NONE',  ( -8.376464375933499795, -79.43904992786433183, -4.482401383029819719 ) ) ;
#40224=CARTESIAN_POINT ( 'NONE',  ( -1.243323288595322929, -79.18571856227184469, 9.501473710774742898 ) ) ;
#40248=CARTESIAN_POINT ( 'NONE',  ( 5.838193839761705917, -77.47708333333333997, -7.596835002782701629 ) ) ;
#40268=ORIENTED_EDGE ( 'NONE', *, *, #23501, .T. ) ;
#40287=CARTESIAN_POINT ( 'NONE',  ( 1.488544850709269340, -79.26244586587921503, 9.382635476564523458 ) ) ;
#40288=VERTEX_POINT ( 'NONE', #11515 ) ;
#40301=EDGE_CURVE ( 'NONE', #1747, #10450, #55911, .T. ) ;
#40305=CARTESIAN_POINT ( 'NONE',  ( 8.958556919380020744, -77.77414693750340291, -2.998186813234942072 ) ) ;
#40320=CARTESIAN_POINT ( 'NONE',  ( -9.003615175678740812, -78.92666666666666231, -3.133420343058871627 ) ) ;
#40324=ORIENTED_EDGE ( 'NONE', *, *, #42483, .T. ) ;
#40328=CONICAL_SURFACE ( 'NONE', #44081, 1.099999997157999232, 0.7853981633972997312 ) ;
#40371=CARTESIAN_POINT ( 'NONE',  ( -7.364490753307999960, -77.76266001420199814, 6.575368940700000664 ) ) ;
#40406=CARTESIAN_POINT ( 'NONE',  ( 5.809344757335999532, -79.51591332859899808, 7.547947145431999516 ) ) ;
#40429=CARTESIAN_POINT ( 'NONE',  ( 7.430757984336000099, -77.43352694988499252, 5.911115298933000695 ) ) ;
#40443=VECTOR ( 'NONE', #13999, 1000.000000000000000 ) ;
#40450=CARTESIAN_POINT ( 'NONE',  ( 6.772004377195999680, -77.13018832859900442, -6.844728052047999611 ) ) ;
#40464=CARTESIAN_POINT ( 'NONE',  ( -0.6471704932797999188, -77.95024805011499325, 9.701898969124000516 ) ) ;
#40494=CARTESIAN_POINT ( 'NONE',  ( 2.486604901413172808, -78.54583333333330586, -9.252740428348992907 ) ) ;
#40496=CARTESIAN_POINT ( 'NONE',  ( -3.579650252175000436, -77.53493998579799040, 8.845718151729000667 ) ) ;
#40497=CIRCLE ( 'NONE', #24457, 11.44999999999999929 ) ;
#40505=CARTESIAN_POINT ( 'NONE',  ( -0.6521978219530000231, -78.07341332859900263, 9.777264943591001511 ) ) ;
#40518=CARTESIAN_POINT ( 'NONE',  ( -8.539857470955180219, -79.43608207363838858, -4.162491799772078949 ) ) ;
#40520=CARTESIAN_POINT ( 'NONE',  ( -4.417524307039417231, -79.38740258211193179, -8.447129840749521890 ) ) ;
#40536=CARTESIAN_POINT ( 'NONE',  ( 2.486604901413172364, -78.44583333333333997, -9.252740428348998236 ) ) ;
#40585=CARTESIAN_POINT ( 'NONE',  ( -7.785422980193717812, -79.35104354428872853, 5.443977945005203267 ) ) ;
#40614=EDGE_CURVE ( 'NONE', #10884, #5875, #23982, .T. ) ;
#40620=CARTESIAN_POINT ( 'NONE',  ( -8.597941394714000651, -79.60596001420199741, -4.085545016331000312 ) ) ;
#40627=CARTESIAN_POINT ( 'NONE',  ( 1.133919935544836166, -79.28431342984046637, -9.420845921445170745 ) ) ;
#40628=AXIS2_PLACEMENT_3D ( 'NONE', #21018, #39598, #48757 ) ;
#40640=ORIENTED_EDGE ( 'NONE', *, *, #1134, .T. ) ;
#40647=ORIENTED_EDGE ( 'NONE', *, *, #12904, .T. ) ;
#40671=CARTESIAN_POINT ( 'NONE',  ( -9.405253678352000435, -77.73528667140098491, 2.617502431767999571 ) ) ;
#40691=ORIENTED_EDGE ( 'NONE', *, *, #56640, .T. ) ;
#40711=DIRECTION ( 'NONE',  ( -1.000000000000000000, 0.000000000000000000, 0.000000000000000000 ) ) ;
#40727=CARTESIAN_POINT ( 'NONE',  ( -0.7479529023060000892, -77.68867305011499980, -9.465622776916999825 ) ) ;
#40743=CARTESIAN_POINT ( 'NONE',  ( 7.777253296891999845, -77.24328832859900729, 5.676678302143000288 ) ) ;
#40750=VECTOR ( 'NONE', #16351, 1000.000000000000000 ) ;
#40754=CARTESIAN_POINT ( 'NONE',  ( 8.219513559211000242, -78.80469415034599479, 5.194554602171000290 ) ) ;
#40759=ORIENTED_EDGE ( 'NONE', *, *, #15455, .F. ) ;
#40785=CARTESIAN_POINT ( 'NONE',  ( -9.500000000000000000, -78.39999999999999147, 0.000000000000000000 ) ) ;
#40794=CARTESIAN_POINT ( 'NONE',  ( -9.610781959738998736, -78.61933998579799265, 1.214124111355000091 ) ) ;
#40809=CARTESIAN_POINT ( 'NONE',  ( -5.127834196515462573, -79.47936672015556780, -7.997626843221576465 ) ) ;
#40829=CARTESIAN_POINT ( 'NONE',  ( 4.784380313523556083, -78.46666666666665435, -8.300970689365444244 ) ) ;
#40834=CARTESIAN_POINT ( 'NONE',  ( 5.807838419656999207, -77.32737403538303056, -7.511754867730999763 ) ) ;
#40848=ADVANCED_FACE ( 'NONE', ( #32828 ), #37268, .F. ) ;
#40903=ORIENTED_EDGE ( 'NONE', *, *, #49946, .T. ) ;
#40905=CARTESIAN_POINT ( 'NONE',  ( 9.500000000000000000, -77.14999999999999147, 0.000000000000000000 ) ) ;
#40926=B_SPLINE_CURVE_WITH_KNOTS ( 'NONE', 3,
 ( #10671, #5351, #37218, #41371, #18937, #32777, #19813, #36927, #54659, #37806 ),
 .UNSPECIFIED., .F., .F.,
 ( 4, 2, 2, 2, 4 ),
 ( 0.000000000000000000, 0.2500000000000000000, 0.5000000000000000000, 0.7500000000000000000, 1.000000000000000000 ),
 .UNSPECIFIED. ) ;
#40958=CARTESIAN_POINT ( 'NONE',  ( -5.629566154268999867, -77.14463501420200942, -7.542197886061999590 ) ) ;
#40978=CARTESIAN_POINT ( 'NONE',  ( 9.500000000000000000, -78.64999999999999147, 0.000000000000000000 ) ) ;
#40980=DIRECTION ( 'NONE',  ( -1.000000000000000000, 0.000000000000000000, 0.000000000000000000 ) ) ;
#40996=VERTEX_POINT ( 'NONE', #48467 ) ;
#40998=CARTESIAN_POINT ( 'NONE',  ( 3.013969474723999564, -79.34431332859900010, -8.821166524726999469 ) ) ;
#41000=DIRECTION ( 'NONE',  ( 1.000000000000000000, 0.000000000000000000, 0.000000000000000000 ) ) ;
#41007=ORIENTED_EDGE ( 'NONE', *, *, #22813, .F. ) ;
#41017=CARTESIAN_POINT ( 'NONE',  ( -0.7479529023060000892, -77.74877694988499854, -9.465622776916999825 ) ) ;
#41026=CARTESIAN_POINT ( 'NONE',  ( 8.300970689365438915, -77.59166666666666856, 4.784380313523563188 ) ) ;
#41036=CARTESIAN_POINT ( 'NONE',  ( 2.216541547539999879, -77.23606498579799506, 9.481530790117000507 ) ) ;
#41047=CARTESIAN_POINT ( 'NONE',  ( 9.218641115533358743, -77.00000000000001421, -2.097425539381363446 ) ) ;
#41050=CARTESIAN_POINT ( 'NONE',  ( 4.316051676898999823, -78.84824415034599099, 8.712949996777000550 ) ) ;
#41102=FACE_OUTER_BOUND ( 'NONE', #15740, .T. ) ;
#41122=CARTESIAN_POINT ( 'NONE',  ( -9.391369684923001060, -77.13822403538300421, 1.399863080762999923 ) ) ;
#41144=CARTESIAN_POINT ( 'NONE',  ( -7.596835002782709623, -77.85208333333333997, -5.838193839761696147 ) ) ;
#41155=ORIENTED_EDGE ( 'NONE', *, *, #7953, .T. ) ;
#41176=CARTESIAN_POINT ( 'NONE',  ( 9.091459715836720079, -77.32174693750340566, 2.567140442679551438 ) ) ;
#41183=CARTESIAN_POINT ( 'NONE',  ( -3.063214743671000218, -79.10658667140098999, -9.307899183505000451 ) ) ;
#41198=FACE_OUTER_BOUND ( 'NONE', #51336, .T. ) ;
#41228=CARTESIAN_POINT ( 'NONE',  ( 9.151322089608749266, -79.17128379080990896, 2.562544536898030412 ) ) ;
#41250=VECTOR ( 'NONE', #536, 1000.000000000000000 ) ;
#41252=CARTESIAN_POINT ( 'NONE',  ( 0.7029086986541999149, -77.56231332859900363, 9.627002478265000107 ) ) ;
#41259=CARTESIAN_POINT ( 'NONE',  ( 0.000000000000000000, -74.70999999999999375, 0.000000000000000000 ) ) ;
#41265=AXIS2_PLACEMENT_3D ( 'NONE', #2852, #56581, #48884 ) ;
#41282=CARTESIAN_POINT ( 'NONE',  ( -0.9736830274145173991, -76.99999999999998579, 9.250386169343817855 ) ) ;
#41306=CARTESIAN_POINT ( 'NONE',  ( 4.574312611392000072, -77.40494805011499579, 8.320643751074999983 ) ) ;
#41315=ORIENTED_EDGE ( 'NONE', *, *, #56415, .T. ) ;
#41316=CARTESIAN_POINT ( 'NONE',  ( -5.838193839761721016, -77.72708333333332575, 7.596835002782687418 ) ) ;
#41331=VERTEX_POINT ( 'NONE', #16734 ) ;
#41336=CARTESIAN_POINT ( 'NONE',  ( 7.722022491113547993, -76.99999999999998579, 5.250591757671347004 ) ) ;
#41371=CARTESIAN_POINT ( 'NONE',  ( -8.536051545334721879, -79.70833333333069959, -3.797199644221384229 ) ) ;
#41372=VERTEX_POINT ( 'NONE', #30290 ) ;
#41374=CARTESIAN_POINT ( 'NONE',  ( -9.927618387633998509, -77.89028998579800600, -1.374747298418999897 ) ) ;
#41385=ORIENTED_EDGE ( 'NONE', *, *, #44501, .T. ) ;
#41417=CARTESIAN_POINT ( 'NONE',  ( 2.858407197969000002, -77.00000000000000000, 8.797272775729998884 ) ) ;
#41439=CARTESIAN_POINT ( 'NONE',  ( -4.784380313523538319, -77.88333333333332575, -8.300970689365453126 ) ) ;
#41454=FACE_OUTER_BOUND ( 'NONE', #5549, .T. ) ;
#41488=CARTESIAN_POINT ( 'NONE',  ( -2.362630825376999866, -79.54861332859900358, -9.447900677770000755 ) ) ;
#41501=CARTESIAN_POINT ( 'NONE',  ( -9.554796630153999715, -79.63025194988500743, -0.02401403847836000235 ) ) ;
#41536=AXIS2_PLACEMENT_3D ( 'NONE', #24420, #42434, #33551 ) ;
#41577=CARTESIAN_POINT ( 'NONE',  ( -7.591546392047000325, -79.74471332859900485, -5.752267283136999865 ) ) ;
#41578=DIRECTION ( 'NONE',  ( 0.000000000000000000, 1.000000000000000000, 0.000000000000000000 ) ) ;
#41587=CARTESIAN_POINT ( 'NONE',  ( 0.000000000000000000, -75.10000000284179578, -7.200000000000000178 ) ) ;
#41593=VERTEX_POINT ( 'NONE', #26731 ) ;
#41598=CARTESIAN_POINT ( 'NONE',  ( 9.136202122873999798, -77.40200194988500471, 2.585973524422000125 ) ) ;
#41606=ORIENTED_EDGE ( 'NONE', *, *, #3957, .T. ) ;
#41624=FACE_OUTER_BOUND ( 'NONE', #3609, .T. ) ;
#41661=CARTESIAN_POINT ( 'NONE',  ( 0.3023719455682368218, -77.77249999999999375, 9.537307262745171599 ) ) ;
#41700=CARTESIAN_POINT ( 'NONE',  ( -9.601739433208001273, -79.20275584965399673, -1.533141744029000053 ) ) ;
#41725=CARTESIAN_POINT ( 'NONE',  ( 0.000000000000000000, -76.00000000000000000, 0.000000000000000000 ) ) ;
#41747=CARTESIAN_POINT ( 'NONE',  ( -3.133069020688000084, -79.42036001420198943, -9.520158728599000142 ) ) ;
#41761=CARTESIAN_POINT ( 'NONE',  ( -9.444256657865821580, -77.54794693750339718, 0.2255349141366999877 ) ) ;
#41766=CARTESIAN_POINT ( 'NONE',  ( -5.485200302047999799, -78.64776001420199236, -7.984597978739000901 ) ) ;
#41785=CARTESIAN_POINT ( 'NONE',  ( -2.410095898663000114, -79.33801332859898992, 9.435914216412999878 ) ) ;
#41787=DIRECTION ( 'NONE',  ( 0.000000000000000000, 1.000000000000000000, 0.000000000000000000 ) ) ;
#41794=CARTESIAN_POINT ( 'NONE',  ( 6.479078291783999966, -79.31435194988499404, -7.022474634662000170 ) ) ;
#41802=DIRECTION ( 'NONE',  ( 0.000000000000000000, -0.7071067811866525998, -0.7071067811864425456 ) ) ;
#41806=DIRECTION ( 'NONE',  ( 3.655298286142000429E-11, 1.000000000000000000, -1.590757977788000024E-09 ) ) ;
#41807=EDGE_LOOP ( 'NONE', ( #12313, #5911, #35535, #38316, #48707, #26809, #29233, #52238, #2324 ) ) ;
#41814=VERTEX_POINT ( 'NONE', #9667 ) ;
#41826=CARTESIAN_POINT ( 'NONE',  ( -9.199999999968001774, -80.60000000003199716, 3.388760884947000060E-10 ) ) ;
#41829=FACE_OUTER_BOUND ( 'NONE', #6607, .T. ) ;
#41833=CARTESIAN_POINT ( 'NONE',  ( 9.381339102657999973, -77.31428501420199950, -0.7531566933248999840 ) ) ;
#41836=CARTESIAN_POINT ( 'NONE',  ( -4.784380313523580064, -77.21666666666669698, 8.300970689365431809 ) ) ;
#41838=CARTESIAN_POINT ( 'NONE',  ( -7.200293548019001122, -77.63511332859900449, 6.428765836700999436 ) ) ;
#41841=CARTESIAN_POINT ( 'NONE',  ( 8.803297119250066416, -77.11875000000000568, -3.648104604236618087 ) ) ;
#41867=EDGE_CURVE ( 'NONE', #44850, #45023, #28884, .T. ) ;
#41890=CARTESIAN_POINT ( 'NONE',  ( -9.204193785523999694, -77.02959415034598578, -2.332437886131999871 ) ) ;
#41946=CARTESIAN_POINT ( 'NONE',  ( -9.185997767857138285, -77.00000000000001421, 1.529051226933332952 ) ) ;
#41955=CARTESIAN_POINT ( 'NONE',  ( 6.055527902613000002, -77.71999999999999886, 7.319875806370000682 ) ) ;
#41959=CARTESIAN_POINT ( 'NONE',  ( -9.486322910027237043, -79.39542840225620068, 0.5339199459016039651 ) ) ;
#41979=DIRECTION ( 'NONE',  ( 0.000000000000000000, 0.000000000000000000, -1.000000000000000000 ) ) ;
#41984=ORIENTED_EDGE ( 'NONE', *, *, #30468, .F. ) ;
#42000=FACE_OUTER_BOUND ( 'NONE', #32132, .T. ) ;
#42020=CARTESIAN_POINT ( 'NONE',  ( -9.199999999999999289, -79.79999999999999716, 0.000000000000000000 ) ) ;
#42022=CARTESIAN_POINT ( 'NONE',  ( 9.500000000000000000, -78.04999999999999716, 0.000000000000000000 ) ) ;
#42039=CARTESIAN_POINT ( 'NONE',  ( 4.634228027295999475, -78.15741001420200007, 8.886345528036001085 ) ) ;
#42056=CARTESIAN_POINT ( 'NONE',  ( -7.483407197968000801, -77.00000000000000000, 5.437013583706000297 ) ) ;
#42060=CARTESIAN_POINT ( 'NONE',  ( -8.963686800021001488, -79.03971001420200082, 3.673354096997999640 ) ) ;
#42086=CARTESIAN_POINT ( 'NONE',  ( 2.013632425233999879, -78.29159514476064885, -9.512575055159999238 ) ) ;
#42090=CARTESIAN_POINT ( 'NONE',  ( 8.395992668097999712, -79.35954805011499502, 4.560928606276999808 ) ) ;
#42095=VERTEX_POINT ( 'NONE', #48806 ) ;
#42096=EDGE_CURVE ( 'NONE', #50093, #37236, #17324, .T. ) ;
#42117=CARTESIAN_POINT ( 'NONE',  ( 0.000000000000000000, -75.00000000000000000, 0.000000000000000000 ) ) ;
#42130=DIRECTION ( 'NONE',  ( 0.000000000000000000, 0.000000000000000000, -1.000000000000000000 ) ) ;
#42144=CARTESIAN_POINT ( 'NONE',  ( -9.646692012709999986, -78.55994805011499693, 1.218660606027000215 ) ) ;
#42170=EDGE_CURVE ( 'NONE', #1747, #13828, #3855, .T. ) ;
#42181=CARTESIAN_POINT ( 'NONE',  ( -8.268101562183998610, -77.17093998579798608, -4.764359567075000079 ) ) ;
#42189=CARTESIAN_POINT ( 'NONE',  ( -7.591316436381999821, -77.06111915034600202, -5.703451837412999659 ) ) ;
#42193=CARTESIAN_POINT ( 'NONE',  ( -3.040079553448159722, -79.14882913613843129, -9.237600482237251498 ) ) ;
#42207=FACE_OUTER_BOUND ( 'NONE', #15293, .T. ) ;
#42218=B_SPLINE_CURVE_WITH_KNOTS ( 'NONE', 3,
 ( #43799, #6904, #24912, #2485, #20488, #38485, #44657, #13050, #44951, #13643, #4799, #27212, #22207, #52935, #57935, #4211, #53218, #34904, #35780, #31638, #53809, #8635, #8342, #35478, #17794, #26621, #53509, #40518, #49681, #13345, #31342, #9226, #49384, #17198, #48509, #401, #40218, #22800, #8932, #45250, #58229, #12766, #4506, #17491, #31048, #22508, #12483, #26921, #3625, #44076, #49083, #35186, #36082, #111, #40809, #30483, #26051, #18089, #8056, #54101, #21630, #39635, #57643, #30762 ),
 .UNSPECIFIED., .F., .F.,
 ( 4, 2, 2, 1, 2, 2, 1, 1, 1, 2, 1, 1, 2, 2, 1, 2, 2, 2, 1, 1, 1, 2, 2, 2, 2, 2, 2, 2, 2, 2, 2, 2, 1, 2, 2, 1, 2, 4 ),
 ( 0.7213274189558753768, 0.7387444552711300849, 0.7474529734287574945, 0.7496301029681643469, 0.7499022441605901479, 0.7501743853530160600, 0.7507186677378677730, 0.7518072325075711992, 0.7561614915863849040, 0.7735785279016396121, 0.7822870460592670216, 0.7844641755986738740, 0.7855527403683773002, 0.7860970227532290133, 0.7866413051380807264, 0.7909955642168944312, 0.8084126005321492503, 0.8171211186897766598, 0.8192982482291834012, 0.8203868129988868274, 0.8209310953837385405, 0.8212032365761644526, 0.8214753777685903646, 0.8258296368474051796, 0.8606637094779239217, 0.8780807457931834037, 0.8867892639508130337, 0.8911435230296278487, 0.8933206525690353672, 0.8954977821084427747, 0.9303318547389628490, 0.9390403728965928121, 0.9433946319754078491, 0.9455717615148153676, 0.9466603262845191269, 0.9477488910542228862, 0.9651659273694819241, 1.000000000000000000 ),
 .UNSPECIFIED. ) ;
#42256=CARTESIAN_POINT ( 'NONE',  ( -9.144741847372999999, -78.41288998579800307, -4.101371784086000005 ) ) ;
#42260=CARTESIAN_POINT ( 'NONE',  ( -9.040761882004836991, -79.37487198799524890, 2.917428640528126671 ) ) ;
#42268=VERTEX_POINT ( 'NONE', #45192 ) ;
#42293=CARTESIAN_POINT ( 'NONE',  ( -7.401612602209000968, -79.24630584965400715, -6.305503003149000030 ) ) ;
#42329=ADVANCED_FACE ( 'NONE', ( #41624 ), #1204, .T. ) ;
#42337=AXIS2_PLACEMENT_3D ( 'NONE', #23007, #24174, #23585 ) ;
#42346=CARTESIAN_POINT ( 'NONE',  ( 7.128677745341877703, -77.70833333333332860, 6.432089047655187741 ) ) ;
#42357=CARTESIAN_POINT ( 'NONE',  ( 2.227885729735000098, -79.15013667140100040, -9.542051086884001165 ) ) ;
#42365=DIRECTION ( 'NONE',  ( 0.000000000000000000, 1.000000000000000000, 0.000000000000000000 ) ) ;
#42377=CARTESIAN_POINT ( 'NONE',  ( -2.389266123960000154, -79.48483998579800414, -9.554412305752000734 ) ) ;
#42378=DIRECTION ( 'NONE',  ( -1.000000000000000000, 0.000000000000000000, 0.000000000000000000 ) ) ;
#42382=CARTESIAN_POINT ( 'NONE',  ( 6.669449228234999971, -78.33514514476064505, -7.075468016816000016 ) ) ;
#42386=CARTESIAN_POINT ( 'NONE',  ( 6.479078291783999966, -79.37445584965399803, -7.022474634662000170 ) ) ;
#42406=CARTESIAN_POINT ( 'NONE',  ( 6.204990652802643503, -79.21820937768764281, 7.193542684779512975 ) ) ;
#42415=CARTESIAN_POINT ( 'NONE',  ( 0.000000000000000000, -75.10000000284179578, -7.200000000000000178 ) ) ;
#42418=EDGE_CURVE ( 'NONE', #14353, #23790, #50496, .T. ) ;
#42422=FACE_OUTER_BOUND ( 'NONE', #9319, .T. ) ;
#42434=DIRECTION ( 'NONE',  ( 0.000000000000000000, 1.000000000000000000, 0.000000000000000000 ) ) ;
#42483=EDGE_CURVE ( 'NONE', #49808, #1317, #32743, .T. ) ;
#42485=CARTESIAN_POINT ( 'NONE',  ( 0.000000000000000000, -76.79999999999999716, 0.000000000000000000 ) ) ;
#42486=CARTESIAN_POINT ( 'NONE',  ( 1.134100835125040119, -79.18344744587857065, -9.422324300646277351 ) ) ;
#42504=DIRECTION ( 'NONE',  ( 0.000000000000000000, -1.000000000000000000, 0.000000000000000000 ) ) ;
#42524=B_SPLINE_CURVE_WITH_KNOTS ( 'NONE', 3,
 ( #39640, #53224, #44662, #13648, #26344, #22213, #44362, #3915, #13055, #31054, #40224, #58235, #53814, #28092, #55556, #6248, #50854, #51146, #5960, #9817, #5665, #46431 ),
 .UNSPECIFIED., .F., .F.,
 ( 4, 2, 2, 2, 2, 2, 2, 2, 2, 2, 4 ),
 ( 0.3902582218033504580, 0.4664759440779315813, 0.5426936663525125937, 0.5808025274898032109, 0.6189113886270938281, 0.6951291109016750625, 0.7713468331762562968, 0.8475645554508375312, 0.8856734165881281484, 0.9237822777254187656, 1.000000000000000000 ),
 .UNSPECIFIED. ) ;
#42542=CARTESIAN_POINT ( 'NONE',  ( -9.500000000000000000, -77.89999999999999147, 0.000000000000000000 ) ) ;
#42546=CARTESIAN_POINT ( 'NONE',  ( -9.037065544638657855, -79.37477492731599682, 2.928856757568816693 ) ) ;
#42548=B_SPLINE_CURVE_WITH_KNOTS ( 'NONE', 3,
 ( #27136, #27433, #8854, #41026, #32147, #54610, #50187, #26844, #9732, #46059, #36001, #23309, #41316, #44873, #901, #18882, #32434, #36878 ),
 .UNSPECIFIED., .F., .F.,
 ( 4, 2, 2, 2, 2, 2, 2, 2, 4 ),
 ( 0.000000000000000000, 0.1250000000000000278, 0.2500000000000000555, 0.3750000000000001110, 0.5000000000000001110, 0.6250000000000001110, 0.7500000000000002220, 0.8750000000000001110, 1.000000000000000000 ),
 .UNSPECIFIED. ) ;
#42628=CARTESIAN_POINT ( 'NONE',  ( -3.063214743671000218, -79.29281332859899578, -9.307899183505000451 ) ) ;
#42630=ORIENTED_EDGE ( 'NONE', *, *, #30277, .F. ) ;
#42645=CARTESIAN_POINT ( 'NONE',  ( 9.557721383756000222, -78.17181332859900067, -2.621152531184999912 ) ) ;
#42652=CARTESIAN_POINT ( 'NONE',  ( 3.938171349113054998, -79.27666666666658557, -8.369041066855391620 ) ) ;
#42663=CARTESIAN_POINT ( 'NONE',  ( -8.916572348234000245, -79.34443998579800450, 4.182142589683000011 ) ) ;
#42669=CARTESIAN_POINT ( 'NONE',  ( -5.600962501325999376, -78.07384514476065362, 7.948110234177999445 ) ) ;
#42673=CARTESIAN_POINT ( 'NONE',  ( -6.090475762158000350, -79.62015584965399739, 7.362120511650999788 ) ) ;
#42677=CARTESIAN_POINT ( 'NONE',  ( 2.486604901413133728, -77.25416666666667709, 9.252740428349007118 ) ) ;
#42693=CARTESIAN_POINT ( 'NONE',  ( 5.930197972290384811, -79.22128088774034893, 7.423945719049496184 ) ) ;
#42709=DIRECTION ( 'NONE',  ( 1.000000000000000000, 0.000000000000000000, 0.000000000000000000 ) ) ;
#42715=CARTESIAN_POINT ( 'NONE',  ( -9.500000000000007105, -77.28958333333333997, 1.243547092045919733 ) ) ;
#42725=FACE_OUTER_BOUND ( 'NONE', #44481, .T. ) ;
#42753=CIRCLE ( 'NONE', #52191, 6.100000000000000533 ) ;
#42767=CARTESIAN_POINT ( 'NONE',  ( -1.267348307942000041, -77.24373998579798695, -9.458036467157000970 ) ) ;
#42773=CARTESIAN_POINT ( 'NONE',  ( 7.092659876394000307, -77.81771915034599374, 6.312768414564000174 ) ) ;
#42786=CARTESIAN_POINT ( 'NONE',  ( -8.300970689365467337, -78.85833333333332007, 4.784380313523513450 ) ) ;
#42822=CARTESIAN_POINT ( 'NONE',  ( -8.919445846190019012, -77.00000000000001421, 2.652912942031755872 ) ) ;
#42830=VERTEX_POINT ( 'NONE', #43370 ) ;
#42858=CARTESIAN_POINT ( 'NONE',  ( 0.000000000000000000, -78.79999999980499581, 0.000000000000000000 ) ) ;
#42897=CARTESIAN_POINT ( 'NONE',  ( 5.896171905175000560, -77.96999999999999886, 7.127247495676000355 ) ) ;
#42903=ORIENTED_EDGE ( 'NONE', *, *, #49913, .T. ) ;
#42918=CARTESIAN_POINT ( 'NONE',  ( -7.662730551410999347, -78.63956332859899589, 6.107448752912000067 ) ) ;
#42937=CARTESIAN_POINT ( 'NONE',  ( -3.098141882180000195, -79.04281332859899578, -9.414028956051998520 ) ) ;
#42939=EDGE_CURVE ( 'NONE', #52539, #54974, #23471, .T. ) ;
#42964=CARTESIAN_POINT ( 'NONE',  ( 9.722066209057999231, -78.90129514476063832, 0.1588365413100999990 ) ) ;
#42967=CARTESIAN_POINT ( 'NONE',  ( 8.857115352654000517, -79.28934805011499520, -3.584237475251999872 ) ) ;
#42968=FACE_OUTER_BOUND ( 'NONE', #44321, .T. ) ;
#42984=CARTESIAN_POINT ( 'NONE',  ( 4.854244445426996180, -79.23213983034467844, 8.180124833994572242 ) ) ;
#42992=CARTESIAN_POINT ( 'NONE',  ( 5.292225205187681247, -79.72180290446119955, -7.854116158959713268 ) ) ;
#43001=DIRECTION ( 'NONE',  ( -1.000000000000000000, 0.000000000000000000, 0.000000000000000000 ) ) ;
#43017=CARTESIAN_POINT ( 'NONE',  ( -9.199999999968001774, -80.60000000003199716, 3.388760884947000060E-10 ) ) ;
#43061=CARTESIAN_POINT ( 'NONE',  ( 8.256620083228000340, -77.21874415034599792, -4.688888258373000717 ) ) ;
#43073=CARTESIAN_POINT ( 'NONE',  ( 5.131017344144000347, -78.15092668086899153, 8.166481637765999224 ) ) ;
#43096=VERTEX_POINT ( 'NONE', #25513 ) ;
#43152=FILL_AREA_STYLE ('',( #16568 ) ) ;
#43164=CARTESIAN_POINT ( 'NONE',  ( -9.646692012709999986, -78.68015584965399967, 1.218660606027000215 ) ) ;
#43194=ORIENTED_EDGE ( 'NONE', *, *, #29959, .T. ) ;
#43205=CARTESIAN_POINT ( 'NONE',  ( 6.533310722863999942, -79.37991332859898819, -6.649273783659000792 ) ) ;
#43208=ORIENTED_EDGE ( 'NONE', *, *, #25617, .T. ) ;
#43221=B_SPLINE_CURVE_WITH_KNOTS ( 'NONE', 3,
 ( #42542, #18940, #2109, #20109, #55830, #19230, #38100, #5355, #32199, #32488, #5638, #5932, #41661, #55237, #28653, #50825, #23937, #41955 ),
 .UNSPECIFIED., .F., .F.,
 ( 4, 2, 2, 2, 2, 2, 2, 2, 4 ),
 ( 0.000000000000000000, 0.1250000000000000000, 0.2500000000000000000, 0.3750000000000000000, 0.5000000000000000000, 0.6250000000000000000, 0.7500000000000000000, 0.8750000000000000000, 1.000000000000000000 ),
 .UNSPECIFIED. ) ;
#43223=CARTESIAN_POINT ( 'NONE',  ( 9.449971683680001178, -78.23558667140099487, -2.591602768458999950 ) ) ;
#43233=CARTESIAN_POINT ( 'NONE',  ( 4.044903269867999640, -79.46000000000000796, -8.595856998426999240 ) ) ;
#43247=EDGE_CURVE ( 'NONE', #41372, #57123, #10425, .T. ) ;
#43250=EDGE_CURVE ( 'NONE', #45676, #2820, #2164, .T. ) ;
#43271=EDGE_LOOP ( 'NONE', ( #14646, #42903, #18792, #24309 ) ) ;
#43273=CARTESIAN_POINT ( 'NONE',  ( 2.624138108766170152, -79.25253984762679238, 9.130854755080981988 ) ) ;
#43274=B_SPLINE_SURFACE_WITH_KNOTS ( 'NONE', 3, 3, ( 
 ( #50619, #36725, #37600, #41747, #10757, #37017, #45902, #55916, #5433, #15467, #29035, #24324, #28145, #33457, #1039, #1906, #19024, #55031, #55322, #14577, #19900, #47074, #6602, #32571, #37306, #14866, #752, #32863, #10456, #46492, #6016, #24025, #42039, #1608, #48226 ),
 ( #25764, #16623, #12193, #11906, #16342, #7474, #20761, #21047, #38762, #29314, #11627, #30176, #34893, #52922, #21330, #56204, #7183, #47363, #48500, #6895, #2475, #2193, #57348, #24900, #57063, #25183, #39048, #3336, #12470, #34607, #16913, #7760, #16046, #29885, #30474 ),
 ( #43205, #24614, #43784, #42628, #3051, #20478, #33748, #34030, #20191, #2762, #38474, #51786, #39342, #56779, #38183, #15751, #11336, #52637, #42918, #56492, #52069, #29601, #47655, #34319, #52355, #47943, #25471, #43491, #100, #26909, #17780, #40505, #44065, #58217, #8621 ),
 ( #18075, #36069, #8043, #39909, #17480, #3613, #44939, #31036, #54090, #3896, #21618, #4784, #53207, #22786, #18365, #31626, #53495, #40794, #39623, #27199, #35175, #17186, #22195, #8330, #9212, #4496, #389, #57631, #21899, #40207, #36359, #30751, #13038, #4198, #12755 ) ),
 .UNSPECIFIED., .F., .F., .F.,
 ( 4, 4 ),
 ( 4, 1, 1, 1, 1, 1, 1, 1, 1, 1, 1, 1, 1, 1, 1, 1, 1, 1, 1, 1, 1, 1, 1, 1, 1, 1, 1, 1, 1, 1, 1, 1, 4 ),
 ( -0.1377334280162000046, 1.137733428016000081 ),
 ( -0.02000000000000000042, 0.01250000000000000069, 0.04499999999999999833, 0.07749999999999999944, 0.1100000000000000006, 0.1424999999999999878, 0.1749999999999999889, 0.2074999999999999900, 0.2399999999999999911, 0.2725000000000000200, 0.3049999999999999933, 0.3375000000000000222, 0.3699999999999999956, 0.4025000000000000244, 0.4349999999999999978, 0.4675000000000000266, 0.5000000000000000000, 0.5324999999999999734, 0.5649999999999999467, 0.5975000000000000311, 0.6300000000000000044, 0.6624999999999999778, 0.6949999999999999512, 0.7275000000000000355, 0.7600000000000000089, 0.7924999999999999822, 0.8249999999999999556, 0.8575000000000000400, 0.8900000000000000133, 0.9224999999999999867, 0.9549999999999999600, 0.9875000000000000444, 1.020000000000000018 ),
 .UNSPECIFIED. ) ;
#43321=CARTESIAN_POINT ( 'NONE',  ( 1.199999995321999968, -75.00000000467838390, 7.200000027511999079 ) ) ;
#43346=CARTESIAN_POINT ( 'NONE',  ( -7.402774007061660555, -79.10527913613843509, -6.306492414806010416 ) ) ;
#43352=CARTESIAN_POINT ( 'NONE',  ( -5.838193839761687265, -77.97291666666664867, -7.596835002782715840 ) ) ;
#43370=CARTESIAN_POINT ( 'NONE',  ( 7.685661446562000343, -77.00000000000000000, -5.583959896779000509 ) ) ;
#43386=CARTESIAN_POINT ( 'NONE',  ( 5.941822435829999804, -79.64346001420200594, 7.720072325980000372 ) ) ;
#43440=CARTESIAN_POINT ( 'NONE',  ( 0.000000000000000000, -78.79999999980499581, -5.599999999950999729 ) ) ;
#43445=CARTESIAN_POINT ( 'NONE',  ( 6.482950081930999531, -79.31685194988499177, -6.598019266050999754 ) ) ;
#43462=EDGE_CURVE ( 'NONE', #41593, #54974, #48892, .T. ) ;
#43491=CARTESIAN_POINT ( 'NONE',  ( -7.589275504201999922, -78.24761332859900165, -6.198488971763000066 ) ) ;
#43510=CARTESIAN_POINT ( 'NONE',  ( -3.365558374102000094, -78.40978667140099390, 9.202792326454000360 ) ) ;
#43515=CARTESIAN_POINT ( 'NONE',  ( -9.500000000000000000, -78.79999999999999716, 0.000000000000000000 ) ) ;
#43526=AXIS2_PLACEMENT_3D ( 'NONE', #45889, #10156, #14564 ) ;
#43551=ORIENTED_EDGE ( 'NONE', *, *, #30419, .F. ) ;
#43559=CARTESIAN_POINT ( 'NONE',  ( -5.911019111731017794, -79.32841036596610707, 7.438469953604046836 ) ) ;
#43579=CARTESIAN_POINT ( 'NONE',  ( -1.642669681205999765, -77.61808667140098805, -9.377281606960000460 ) ) ;
#43580=CONICAL_SURFACE ( 'NONE', #11519, 11.54999999996000071, 0.7853981633972997312 ) ;
#43622=ORIENTED_EDGE ( 'NONE', *, *, #11339, .F. ) ;
#43637=CARTESIAN_POINT ( 'NONE',  ( -9.319010416584660561, -79.68098958332934956, 1.219003400097848910 ) ) ;
#43684=CARTESIAN_POINT ( 'NONE',  ( 2.815219788740999984, -79.60828667140098958, 9.212769588529999609 ) ) ;
#43696=ADVANCED_FACE ( 'NONE', ( #70 ), #53181, .T. ) ;
#43742=CARTESIAN_POINT ( 'NONE',  ( 5.279327442448000340, -79.24223138344899553, -7.780650776298999816 ) ) ;
#43766=DIRECTION ( 'NONE',  ( 0.000000000000000000, 0.000000000000000000, -1.000000000000000000 ) ) ;
#43780=ORIENTED_EDGE ( 'NONE', *, *, #31115, .T. ) ;
#43784=CARTESIAN_POINT ( 'NONE',  ( 2.227885729735000098, -79.33636332859900619, -9.542051086884001165 ) ) ;
#43799=CARTESIAN_POINT ( 'NONE',  ( -9.500094076791862463, -79.39994338716823563, -4.328536937075411965E-07 ) ) ;
#43808=DIRECTION ( 'NONE',  ( 0.000000000000000000, -1.000000000000000000, 0.000000000000000000 ) ) ;
#43828=CARTESIAN_POINT ( 'NONE',  ( 7.541360678298886455, -79.09749999999999659, -5.846326858574182772 ) ) ;
#43834=AXIS2_PLACEMENT_3D ( 'NONE', #10253, #31789, #49832 ) ;
#43840=CARTESIAN_POINT ( 'NONE',  ( -8.630067035710000667, -79.54514415034600461, -4.100810385846999750 ) ) ;
#43858=CARTESIAN_POINT ( 'NONE',  ( -3.479070826201084543, -79.30455014728846663, 8.840435339296620398 ) ) ;
#43877=DIRECTION ( 'NONE',  ( 0.000000000000000000, -1.000000000000000000, 0.000000000000000000 ) ) ;
#43912=CONICAL_SURFACE ( 'NONE', #53334, 5.199999999809000073, 0.7853981633972997312 ) ;
#43927=CARTESIAN_POINT ( 'NONE',  ( -7.473530895688906384, -79.65494791666267815, 5.742368501771844436 ) ) ;
#43933=CARTESIAN_POINT ( 'NONE',  ( -5.436604004633999843, -77.33488667140099437, -8.108850267457999195 ) ) ;
#43955=CIRCLE ( 'NONE', #27922, 9.199999999999999289 ) ;
#43965=DIRECTION ( 'NONE',  ( -1.000000000000000000, 0.000000000000000000, 0.000000000000000000 ) ) ;
#43985=CARTESIAN_POINT ( 'NONE',  ( -9.061228178001998756, -77.71430584965399646, -2.837532765875999896 ) ) ;
#43986=CIRCLE ( 'NONE', #9096, 5.100000000000000533 ) ;
#44019=CARTESIAN_POINT ( 'NONE',  ( 3.148593469528859767, -77.00000000000000000, 8.707564246707935496 ) ) ;
#44022=CARTESIAN_POINT ( 'NONE',  ( -8.997179024602999675, -79.03899805011499780, 3.687079342327000298 ) ) ;
#44050=AXIS2_PLACEMENT_3D ( 'NONE', #11653, #51811, #11367 ) ;
#44065=CARTESIAN_POINT ( 'NONE',  ( 4.530904210857999992, -78.02986332859900642, 8.688217354640999091 ) ) ;
#44076=CARTESIAN_POINT ( 'NONE',  ( -6.387953794381322936, -79.46628966331279287, -7.041750404545100039 ) ) ;
#44081=AXIS2_PLACEMENT_3D ( 'NONE', #41587, #32126, #28280 ) ;
#44114=B_SPLINE_CURVE_WITH_KNOTS ( 'NONE', 3,
 ( #53857, #54724, #46180, #24004, #41144, #36997, #41439, #19297, #32264, #19882, #5705, #55305, #19005, #55896, #1304, #1024, #45886, #42022 ),
 .UNSPECIFIED., .F., .F.,
 ( 4, 2, 2, 2, 2, 2, 2, 2, 4 ),
 ( 0.000000000000000000, 0.1250000000000000833, 0.2500000000000001665, 0.3750000000000002220, 0.5000000000000002220, 0.6250000000000002220, 0.7500000000000001110, 0.8750000000000001110, 1.000000000000000000 ),
 .UNSPECIFIED. ) ;
#44126=CARTESIAN_POINT ( 'NONE',  ( -4.784380313523580064, -78.71666666666669698, 8.300970689365431809 ) ) ;
#44131=EDGE_LOOP ( 'NONE', ( #9207, #25321 ) ) ;
#44139=CARTESIAN_POINT ( 'NONE',  ( 0.9576858015051188389, -79.26683165706418777, 9.453865573464822702 ) ) ;
#44219=CARTESIAN_POINT ( 'NONE',  ( 3.110024790766000358, -77.40768667140099524, -9.254072701159000047 ) ) ;
#44225=CARTESIAN_POINT ( 'NONE',  ( 6.722974506806673745, -79.33790088530881235, -6.669842186947492202 ) ) ;
#44250=FACE_OUTER_BOUND ( 'NONE', #46624, .T. ) ;
#44268=CARTESIAN_POINT ( 'NONE',  ( 9.136202122873999798, -77.46210584965400869, 2.585973524422000125 ) ) ;
#44273=EDGE_CURVE ( 'NONE', #18472, #41331, #37835, .T. ) ;
#44296=ORIENTED_EDGE ( 'NONE', *, *, #25470, .T. ) ;
#44304=CARTESIAN_POINT ( 'NONE',  ( -8.871933854994999535, -78.72370584965399587, -3.979018739998999354 ) ) ;
#44321=EDGE_LOOP ( 'NONE', ( #57369, #35091, #50693, #57634 ) ) ;
#44337=CARTESIAN_POINT ( 'NONE',  ( 7.275511224484000117, -77.93533998579799515, 6.174641004814999334 ) ) ;
#44353=LINE ( 'NONE', #30760, #24338 ) ;
#44362=CARTESIAN_POINT ( 'NONE',  ( -5.795199452793384332, -79.22747400600979972, 7.554545710430467409 ) ) ;
#44422=CARTESIAN_POINT ( 'NONE',  ( -6.391975584201730065, -79.33365083746186031, 7.030076347870032549 ) ) ;
#44481=EDGE_LOOP ( 'NONE', ( #30640, #38542, #55316, #7464 ) ) ;
#44494=CARTESIAN_POINT ( 'NONE',  ( -9.312500000004000356, -79.68749999999599254, 6.570867420027000168E-10 ) ) ;
#44500=DIRECTION ( 'NONE',  ( -1.000000000000000000, 0.000000000000000000, 0.000000000000000000 ) ) ;
#44501=EDGE_CURVE ( 'NONE', #41372, #50093, #17352, .T. ) ;
#44503=CARTESIAN_POINT ( 'NONE',  ( 0.7189379956714000430, -77.68986001420199727, 9.846538930731000505 ) ) ;
#44519=EDGE_CURVE ( 'NONE', #3012, #23500, #5116, .T. ) ;
#44583=CARTESIAN_POINT ( 'NONE',  ( -8.175152901933000038, -76.92503998579799429, -5.289553387389999806 ) ) ;
#44595=CARTESIAN_POINT ( 'NONE',  ( 9.029734473257063243, -77.00000000000000000, -2.837209596131928802 ) ) ;
#44599=CARTESIAN_POINT ( 'NONE',  ( 9.377128579935000374, -78.29864805011499129, -2.571625947824999869 ) ) ;
#44617=ORIENTED_EDGE ( 'NONE', *, *, #3751, .F. ) ;
#44638=ORIENTED_EDGE ( 'NONE', *, *, #16691, .F. ) ;
#44657=CARTESIAN_POINT ( 'NONE',  ( -9.392562919573798297, -79.41163292977475407, -1.424155904483036084 ) ) ;
#44662=CARTESIAN_POINT ( 'NONE',  ( -9.253333465380869427, -79.27966831068214049, 2.487796638288232831 ) ) ;
#44683=B_SPLINE_CURVE_WITH_KNOTS ( 'NONE', 3,
 ( #15179, #6616, #29048, #33172 ),
 .UNSPECIFIED., .F., .F.,
 ( 4, 4 ),
 ( 0.000000000000000000, 0.2500000082780876598 ),
 .UNSPECIFIED. ) ;
#44713=ORIENTED_EDGE ( 'NONE', *, *, #31074, .T. ) ;
#44722=CARTESIAN_POINT ( 'NONE',  ( -3.386084928587058229, -79.30373914007272163, 8.876438725661222051 ) ) ;
#44753=CARTESIAN_POINT ( 'NONE',  ( -4.418379168946118263, -78.98666666666667879, -8.447563838020446525 ) ) ;
#44755=CARTESIAN_POINT ( 'NONE',  ( 9.613649280381000750, -79.26138667140099869, 0.5442168635241999564 ) ) ;
#44805=CARTESIAN_POINT ( 'NONE',  ( -9.511284522137000152, -77.79906001420199857, 2.647011044820000158 ) ) ;
#44835=CARTESIAN_POINT ( 'NONE',  ( 0.000000000000000000, -80.59999999999999432, -9.199999999999974420 ) ) ;
#44850=VERTEX_POINT ( 'NONE', #39463 ) ;
#44862=EDGE_CURVE ( 'NONE', #37723, #8940, #11457, .T. ) ;
#44873=CARTESIAN_POINT ( 'NONE',  ( -7.596835002782738933, -77.74791666666666856, 5.838193839761661508 ) ) ;
#44885=CARTESIAN_POINT ( 'NONE',  ( -7.445902463126000015, -77.49776332859899242, -6.104824477164000562 ) ) ;
#44894=CARTESIAN_POINT ( 'NONE',  ( 7.551616412536306555, -76.99999999999998579, 5.485893062531241426 ) ) ;
#44896=CARTESIAN_POINT ( 'NONE',  ( -8.918806285220000518, -77.97724415034599588, 3.872830773119999570 ) ) ;
#44920=CARTESIAN_POINT ( 'NONE',  ( 9.199999999999999289, -80.59999999999999432, 0.000000000000000000 ) ) ;
#44923=CARTESIAN_POINT ( 'NONE',  ( 0.000000000000000000, -75.20000000000000284, 0.000000000000000000 ) ) ;
#44931=CARTESIAN_POINT ( 'NONE',  ( 7.965859911057998843, -77.42573998579798911, 5.254112810574000036 ) ) ;
#44937=EDGE_CURVE ( 'NONE', #42095, #53581, #9837, .T. ) ;
#44939=CARTESIAN_POINT ( 'NONE',  ( -8.963686800021001488, -79.09838998579799352, 3.673354096997999640 ) ) ;
#44943=CARTESIAN_POINT ( 'NONE',  ( 8.857589609082554105, -79.26910282387936491, -3.584429394132419677 ) ) ;
#44944=ORIENTED_EDGE ( 'NONE', *, *, #3038, .T. ) ;
#44951=CARTESIAN_POINT ( 'NONE',  ( -9.382670943801374008, -79.41215256169735426, -1.487056722518299345 ) ) ;
#44953=CARTESIAN_POINT ( 'NONE',  ( 2.562649862274036572, -79.44753403950033999, -9.184391689306689699 ) ) ;
#44970=CARTESIAN_POINT ( 'NONE',  ( -9.500000000000000000, -78.29999999999999716, 0.000000000000000000 ) ) ;
#44981=CARTESIAN_POINT ( 'NONE',  ( 4.784380313523556083, -77.46666666666668277, -8.300970689365444244 ) ) ;
#45023=VERTEX_POINT ( 'NONE', #11963 ) ;
#45058=CARTESIAN_POINT ( 'NONE',  ( 5.662870153706999865, -79.74636001420199705, -7.651606806962000462 ) ) ;
#45108=CARTESIAN_POINT ( 'NONE',  ( 3.755238055182999801, -78.09928667140098923, 8.648011040868999189 ) ) ;
#45111=CARTESIAN_POINT ( 'NONE',  ( 9.063334061753160142, -77.12500000000001421, -2.943243628773176024 ) ) ;
#45165=CARTESIAN_POINT ( 'NONE',  ( 1.529609450199000076, -76.99217694988499261, 9.371081266747001592 ) ) ;
#45183=CARTESIAN_POINT ( 'NONE',  ( -9.199999999999999289, -77.00000000000000000, 0.000000000000000000 ) ) ;
#45184=CARTESIAN_POINT ( 'NONE',  ( 0.6679705033387999258, -77.07363832859898878, -9.605423498967001095 ) ) ;
#45192=CARTESIAN_POINT ( 'NONE',  ( 0.000000000000000000, -76.79999999999999716, -5.100000000000001421 ) ) ;
#45228=CARTESIAN_POINT ( 'NONE',  ( 9.252740428349001789, -78.62916666666666288, -2.486604901413144830 ) ) ;
#45229=CARTESIAN_POINT ( 'NONE',  ( 4.106377143637999438, -77.78973998579799343, -8.613842362031000732 ) ) ;
#45240=CARTESIAN_POINT ( 'NONE',  ( 6.723335045862328663, -79.23760275795656582, -6.670198521808291758 ) ) ;
#45250=CARTESIAN_POINT ( 'NONE',  ( -7.196477163768985719, -79.45634548972412858, -6.205214754808124233 ) ) ;
#45295=DIRECTION ( 'NONE',  ( 0.000000000000000000, -1.000000000000000000, 0.000000000000000000 ) ) ;
#45302=CARTESIAN_POINT ( 'NONE',  ( 0.000000000000000000, -80.70000000003399521, 0.000000000000000000 ) ) ;
#45332=DIRECTION ( 'NONE',  ( 0.000000000000000000, 1.000000000000000000, 0.000000000000000000 ) ) ;
#45352=B_SPLINE_CURVE_WITH_KNOTS ( 'NONE', 3,
 ( #17488, #13640, #8631, #18084, #13046, #26917, #36078, #21337, #109, #12479, #26048, #53505, #39917, #57933, #8053, #31044, #3906, #21908 ),
 .UNSPECIFIED., .F., .F.,
 ( 4, 2, 2, 2, 2, 2, 2, 2, 4 ),
 ( 0.000000000000000000, 0.1249999999999999445, 0.2499999999999998890, 0.3749999999999998335, 0.4999999999999997780, 0.6249999999999997780, 0.7499999999999997780, 0.8749999999999997780, 1.000000000000000000 ),
 .UNSPECIFIED. ) ;
#45400=CARTESIAN_POINT ( 'NONE',  ( 9.057366737456000294, -77.34256001420199311, 2.557513664763999994 ) ) ;
#45402=DIRECTION ( 'NONE',  ( 1.000000000000000000, 0.000000000000000000, 0.000000000000000000 ) ) ;
#45436=ORIENTED_EDGE ( 'NONE', *, *, #23726, .F. ) ;
#45438=CARTESIAN_POINT ( 'NONE',  ( 5.743105918089000284, -79.45213998579799863, 7.461884555157999976 ) ) ;
#45441=DIRECTION ( 'NONE',  ( 0.000000000000000000, 1.000000000000000000, 0.000000000000000000 ) ) ;
#45454=ORIENTED_EDGE ( 'NONE', *, *, #16182, .T. ) ;
#45456=CARTESIAN_POINT ( 'NONE',  ( 0.000000000000000000, -80.79999999999999716, 0.000000000000000000 ) ) ;
#45459=CARTESIAN_POINT ( 'NONE',  ( -9.061228178001998756, -77.59409805011499373, -2.837532765875999896 ) ) ;
#45477=CARTESIAN_POINT ( 'NONE',  ( 7.581939418254000529, -77.57536498579798945, -6.109555841837000401 ) ) ;
#45480=EDGE_LOOP ( 'NONE', ( #15311, #45674, #1738, #46332 ) ) ;
#45487=EDGE_CURVE ( 'NONE', #34323, #34669, #44114, .T. ) ;
#45489=CARTESIAN_POINT ( 'NONE',  ( 7.920136950582000068, -77.86314805011500084, 4.778486233528999705 ) ) ;
#45517=LINE ( 'NONE', #54370, #28059 ) ;
#45520=SURFACE_SIDE_STYLE ('',( #52911 ) ) ;
#45526=CARTESIAN_POINT ( 'NONE',  ( 5.657431823768000356, -76.80693998579801018, -7.274622582025999762 ) ) ;
#45536=CARTESIAN_POINT ( 'NONE',  ( 1.814076166948946689, -79.40950282387937875, 9.381557441920369556 ) ) ;
#45571=CARTESIAN_POINT ( 'NONE',  ( -5.597970637881999778, -77.07517403538302858, 7.669424558767000022 ) ) ;
#45637=FACE_OUTER_BOUND ( 'NONE', #14508, .T. ) ;
#45674=ORIENTED_EDGE ( 'NONE', *, *, #52301, .T. ) ;
#45676=VERTEX_POINT ( 'NONE', #44920 ) ;
#45679=CARTESIAN_POINT ( 'NONE',  ( 9.335966200621838240, -79.16452702242366968, 1.759126508296344760 ) ) ;
#45701=CARTESIAN_POINT ( 'NONE',  ( -8.363462758383999329, -77.23471332859898553, -4.819309911362999799 ) ) ;
#45703=CARTESIAN_POINT ( 'NONE',  ( 7.708428212361858378, -77.10000000000000853, -5.602396082758937190 ) ) ;
#45707=EDGE_CURVE ( 'NONE', #2750, #15146, #23502, .T. ) ;
#45733=CARTESIAN_POINT ( 'NONE',  ( -7.195400558141864522, -77.00000000000001421, 5.833420715738014906 ) ) ;
#45736=CARTESIAN_POINT ( 'NONE',  ( -8.559817476595000585, -79.59513998579799932, 3.923328416589000334 ) ) ;
#45738=CARTESIAN_POINT ( 'NONE',  ( 0.000000000000000000, -77.00000000000000000, 0.000000000000000000 ) ) ;
#45741=ORIENTED_EDGE ( 'NONE', *, *, #48818, .T. ) ;
#45757=CARTESIAN_POINT ( 'NONE',  ( 6.214091009702999102, -77.75172305011498963, -7.179311535719000048 ) ) ;
#45775=CARTESIAN_POINT ( 'NONE',  ( -5.824354096285000004, -76.95331498579798790, -7.803164568795000200 ) ) ;
#45786=CARTESIAN_POINT ( 'NONE',  ( 6.948503177820483323, -77.00000000000000000, 6.231838918554943874 ) ) ;
#45810=CARTESIAN_POINT ( 'NONE',  ( -9.318810932414811177, -77.00000000000001421, -0.6804550629738583822 ) ) ;
#45819=CARTESIAN_POINT ( 'NONE',  ( -7.837473280028000033, -78.32578998579799645, 6.246724465767999668 ) ) ;
#45821=ORIENTED_EDGE ( 'NONE', *, *, #29018, .T. ) ;
#45828=DIRECTION ( 'NONE',  ( -1.000000000000000000, 0.000000000000000000, 0.000000000000000000 ) ) ;
#45865=CARTESIAN_POINT ( 'NONE',  ( 8.979348251287998295, -77.92634903538301216, 3.086914251890999328 ) ) ;
#45872=CARTESIAN_POINT ( 'NONE',  ( 5.454964632513748413, -79.75000000000000000, -7.505574818958165473 ) ) ;
#45886=CARTESIAN_POINT ( 'NONE',  ( 9.500000000000005329, -78.03958333333333997, -1.243547092045939939 ) ) ;
#45889=CARTESIAN_POINT ( 'NONE',  ( 0.000000000000000000, 0.000000000000000000, 0.000000000000000000 ) ) ;
#45902=CARTESIAN_POINT ( 'NONE',  ( -9.273838249849999826, -79.28971001420200082, 3.800455380692000062 ) ) ;
#45907=DIRECTION ( 'NONE',  ( 1.000000000000000000, 0.000000000000000000, 0.000000000000000000 ) ) ;
#45925=CARTESIAN_POINT ( 'NONE',  ( 1.892857502466999797, -78.43001001420199714, 9.500437764121999251 ) ) ;
#45941=CARTESIAN_POINT ( 'NONE',  ( 1.869758079914999982, -79.23913998579800477, 9.669518374590998278 ) ) ;
#45951=CARTESIAN_POINT ( 'NONE',  ( -2.317989000404999889, -79.79565584965399694, -9.269382932261999386 ) ) ;
#45975=CARTESIAN_POINT ( 'NONE',  ( -9.499653450934914645, -79.30027302004205580, 1.387647615217423080E-06 ) ) ;
#45989=CARTESIAN_POINT ( 'NONE',  ( -9.186791650646000562, -77.08808501420200798, -2.044400565391000235 ) ) ;
#46007=CARTESIAN_POINT ( 'NONE',  ( 4.044903269867999640, -79.46000000000000796, -8.595856998426999240 ) ) ;
#46030=CARTESIAN_POINT ( 'NONE',  ( 4.070739930424000619, -79.35384666193300518, -8.460094790468001946 ) ) ;
#46048=CARTESIAN_POINT ( 'NONE',  ( -1.269916711065999904, -77.24437694988499459, -9.409822520238998678 ) ) ;
#46059=CARTESIAN_POINT ( 'NONE',  ( -1.243547092045992564, -77.68541666666665435, 9.499999999999994671 ) ) ;
#46066=DIRECTION ( 'NONE',  ( 0.000000000000000000, -1.000000000000000000, 0.000000000000000000 ) ) ;
#46071=B_SPLINE_SURFACE_WITH_KNOTS ( 'NONE', 3, 3, ( 
 ( #55344, #46218, #10476, #14017, #28167, #14598, #42060, #33177, #32885, #50929, #51224, #28462, #18750, #9603, #1927, #41766, #24346, #46511, #6331, #19334, #45925, #9895, #27589, #6035, #23175, #54762, #24044, #10189, #1631, #36745, #19620, #55636, #15187, #10776, #5172 ),
 ( #28754, #36455, #42357, #41183, #1057, #54482, #32015, #773, #14305, #32299, #50345, #27877, #5458, #24633, #20211, #55935, #7492, #7200, #29904, #43510, #38493, #47959, #21065, #43223, #25489, #56798, #15772, #16065, #3070, #38202, #39069, #25204, #24920, #29052, #52086 ),
 ( #16357, #33764, #19920, #42937, #56222, #47091, #34338, #6913, #51802, #37910, #52374, #15485, #2491, #11356, #11927, #33475, #20497, #29334, #51512, #34048, #11072, #2779, #6622, #42645, #2212, #47381, #56509, #11645, #29622, #47676, #20778, #38779, #10370, #36931, #54944 ),
 ( #10087, #15381, #32780, #27776, #55531, #14783, #46404, #50532, #6223, #24238, #14202, #46113, #23648, #9790, #51121, #37221, #42256, #28066, #45819, #10964, #956, #28947, #24527, #37809, #1240, #46989, #50240, #33375, #41374, #23363, #28358, #14495, #51411, #10674, #6517 ) ),
 .UNSPECIFIED., .F., .F., .F.,
 ( 4, 4 ),
 ( 4, 1, 1, 1, 1, 1, 1, 1, 1, 1, 1, 1, 1, 1, 1, 1, 1, 1, 1, 1, 1, 1, 1, 1, 1, 1, 1, 1, 1, 1, 1, 1, 4 ),
 ( -0.1377334280162000046, 1.137733428016000081 ),
 ( -0.02000000000000000042, 0.01250000000000000069, 0.04499999999999999833, 0.07749999999999999944, 0.1100000000000000006, 0.1424999999999999878, 0.1749999999999999889, 0.2074999999999999900, 0.2399999999999999911, 0.2725000000000000200, 0.3049999999999999933, 0.3375000000000000222, 0.3699999999999999956, 0.4025000000000000244, 0.4349999999999999978, 0.4675000000000000266, 0.5000000000000000000, 0.5324999999999999734, 0.5649999999999999467, 0.5975000000000000311, 0.6300000000000000044, 0.6624999999999999778, 0.6949999999999999512, 0.7275000000000000355, 0.7600000000000000089, 0.7924999999999999822, 0.8249999999999999556, 0.8575000000000000400, 0.8900000000000000133, 0.9224999999999999867, 0.9549999999999999600, 0.9875000000000000444, 1.020000000000000018 ),
 .UNSPECIFIED. ) ;
#46076=DIRECTION ( 'NONE',  ( -0.7071067811865474617, 0.7071067811865474617, 1.027168116582069423E-09 ) ) ;
#46094=EDGE_LOOP ( 'NONE', ( #40640, #29204, #17322, #40647 ) ) ;
#46104=CARTESIAN_POINT ( 'NONE',  ( -2.935661446561999899, -77.00000000000000000, -9.035036904803998681 ) ) ;
#46113=CARTESIAN_POINT ( 'NONE',  ( 10.02101539056000057, -78.63063998579799829, 0.1637206938138999757 ) ) ;
#46119=CARTESIAN_POINT ( 'NONE',  ( -9.500135819972072682, -79.39737933951445825, 0.3021342893088184156 ) ) ;
#46121=B_SPLINE_CURVE_WITH_KNOTS ( 'NONE', 3,
 ( #30323, #8774, #35923, #22347, #17335, #35034, #17053, #49225, #48933, #25903, #8475, #57489, #39488, #43927, #4347, #8192, #43637, #44494 ),
 .UNSPECIFIED., .F., .F.,
 ( 4, 2, 2, 2, 2, 2, 2, 2, 4 ),
 ( 0.000000000000000000, 0.1250000000000000000, 0.2500000000000000000, 0.3750000000000000000, 0.5000000000000000000, 0.6250000000000000000, 0.7500000000000000000, 0.8750000000000000000, 1.000000000000000000 ),
 .UNSPECIFIED. ) ;
#46175=CARTESIAN_POINT ( 'NONE',  ( 9.000000000000000000, -80.79999999999999716, 0.000000000000000000 ) ) ;
#46180=CARTESIAN_POINT ( 'NONE',  ( -9.252740428348994683, -77.82083333333332575, -2.486604901413163926 ) ) ;
#46209=CARTESIAN_POINT ( 'NONE',  ( 3.938458446976999205, -79.30999999999998806, -8.369650235310999165 ) ) ;
#46218=CARTESIAN_POINT ( 'NONE',  ( 5.259675013629999896, -79.24294334753599856, -7.751687108632999035 ) ) ;
#46237=CARTESIAN_POINT ( 'NONE',  ( 7.651633708404999901, -79.64221332859899860, -5.680134239085999681 ) ) ;
#46244=CARTESIAN_POINT ( 'NONE',  ( -6.053394164830000257, -79.76055584965399703, -7.392643757108000813 ) ) ;
#46283=CARTESIAN_POINT ( 'NONE',  ( -1.623939766302999965, -77.68186001420198750, -9.270360727776001397 ) ) ;
#46332=ORIENTED_EDGE ( 'NONE', *, *, #15556, .F. ) ;
#46333=CARTESIAN_POINT ( 'NONE',  ( 0.000000000000000000, -75.10000000019110189, -5.199999999809000073 ) ) ;
#46343=CARTESIAN_POINT ( 'NONE',  ( 2.962511214703000384, -77.72019805011500182, -9.021140561863999707 ) ) ;
#46367=DIRECTION ( 'NONE',  ( -1.000000000000000000, 0.000000000000000000, 0.000000000000000000 ) ) ;
#46396=CARTESIAN_POINT ( 'NONE',  ( -7.726716709342911216, -77.00000000000000000, -5.381598819753512508 ) ) ;
#46404=CARTESIAN_POINT ( 'NONE',  ( -9.273838249849999826, -78.84838998579800773, 3.800455380692000062 ) ) ;
#46409=CARTESIAN_POINT ( 'NONE',  ( -8.590227911348797818, -79.36453639063311982, 4.069435271439020951 ) ) ;
#46431=CARTESIAN_POINT ( 'NONE',  ( 9.500000000000000000, -79.04999999999999716, 0.000000000000000000 ) ) ;
#46492=CARTESIAN_POINT ( 'NONE',  ( -9.193055583834000899, -78.28806001420198868, 3.991918584785999702 ) ) ;
#46506=CARTESIAN_POINT ( 'NONE',  ( -4.370596010382554297, -77.46312193750340214, 8.375126287499346844 ) ) ;
#46511=CARTESIAN_POINT ( 'NONE',  ( -9.610781959738998736, -78.56066001420198575, 1.214124111355000091 ) ) ;
#46541=CARTESIAN_POINT ( 'NONE',  ( 5.684029094576000141, -79.74564805011499402, -7.680196531179999120 ) ) ;
#46567=FACE_OUTER_BOUND ( 'NONE', #10627, .T. ) ;
#46577=CARTESIAN_POINT ( 'NONE',  ( -2.654111470047999966, -77.17291001420200303, -9.029532749234000732 ) ) ;
#46595=CARTESIAN_POINT ( 'NONE',  ( -8.918806285220000518, -78.03734805011499986, 3.872830773119999570 ) ) ;
#46624=EDGE_LOOP ( 'NONE', ( #3566, #50531, #19422, #17320, #28976, #11820 ) ) ;
#46634=CARTESIAN_POINT ( 'NONE',  ( -4.802567994450000377, -77.09264415034600404, -8.191018798270000900 ) ) ;
#46639=CARTESIAN_POINT ( 'NONE',  ( 3.441702665804598382, -77.89481086934992504, 8.844266313550066982 ) ) ;
#46756=DIRECTION ( 'NONE',  ( 0.000000000000000000, -1.000000000000000000, 0.000000000000000000 ) ) ;
#46757=CARTESIAN_POINT ( 'NONE',  ( 9.199999999968001774, -80.60000000003199716, -3.388768808660000233E-10 ) ) ;
#46760=FACE_OUTER_BOUND ( 'NONE', #1499, .T. ) ;
#46773=ORIENTED_EDGE ( 'NONE', *, *, #19222, .T. ) ;
#46781=ORIENTED_EDGE ( 'NONE', *, *, #50020, .T. ) ;
#46784=SHAPE_DEFINITION_REPRESENTATION ( #47926, #1422 ) ;
#46800=CARTESIAN_POINT ( 'NONE',  ( 2.150476488323003199, -77.40657193750340070, 9.198929323063223862 ) ) ;
#46809=CARTESIAN_POINT ( 'NONE',  ( 9.500000000000000000, -78.64999999999999147, 0.000000000000000000 ) ) ;
#46823=CARTESIAN_POINT ( 'NONE',  ( -8.796272286055000222, -79.47841332859898955, -4.179787317773000943 ) ) ;
#46827=CARTESIAN_POINT ( 'NONE',  ( -3.039602602085999639, -79.24969514476062216, -9.236151215514999180 ) ) ;
#46831=CARTESIAN_POINT ( 'NONE',  ( 5.684029094576000141, -79.86585584965399676, -7.680196531179999120 ) ) ;
#46835=CARTESIAN_POINT ( 'NONE',  ( -7.596835002782739821, -77.34791666666667709, 5.838193839761659731 ) ) ;
#46849=CARTESIAN_POINT ( 'NONE',  ( 9.019879307700605864, -79.17500127585684311, 2.981309166188937265 ) ) ;
#46876=PLANE ( 'NONE',  #41536 ) ;
#46932=CARTESIAN_POINT ( 'NONE',  ( -8.873325971494777420, -78.58267913613843803, -3.979643097409233832 ) ) ;
#46989=CARTESIAN_POINT ( 'NONE',  ( 2.075550720420999973, -78.02093998579799461, -9.805082477504999616 ) ) ;
#46994=CARTESIAN_POINT ( 'NONE',  ( -9.471485474656741843, -79.39369676562593270, 0.7342151353995368668 ) ) ;
#47025=VECTOR ( 'NONE', #6546, 1000.000000000000000 ) ;
#47027=CARTESIAN_POINT ( 'NONE',  ( 8.219513559211000242, -78.98500584965400151, 5.194554602171000290 ) ) ;
#47055=DIRECTION ( 'NONE',  ( 1.000000000000000000, 0.000000000000000000, 0.000000000000000000 ) ) ;
#47074=CARTESIAN_POINT ( 'NONE',  ( 6.786979366286999493, -78.63646001420198672, 7.374582364394999701 ) ) ;
#47091=CARTESIAN_POINT ( 'NONE',  ( -9.786657985941999982, -78.95571332859898916, -1.562668305794999934 ) ) ;
#47125=CARTESIAN_POINT ( 'NONE',  ( 5.645287065787000458, -79.45475194988499368, 7.708789581145000014 ) ) ;
#47129=CARTESIAN_POINT ( 'NONE',  ( -5.148784662568076406E-06, -79.56241750339395935, -9.437165819784945953 ) ) ;
#47141=CARTESIAN_POINT ( 'NONE',  ( 7.677756733616925011, -79.19981116400037990, 5.594508313773394192 ) ) ;
#47163=CARTESIAN_POINT ( 'NONE',  ( 4.784380313523521444, -77.13333333333332575, 8.300970689365463784 ) ) ;
#47167=ADVANCED_FACE ( 'NONE', ( #101 ), #18076, .F. ) ;
#47199=EDGE_CURVE ( 'NONE', #43096, #11325, #1213, .T. ) ;
#47211=CARTESIAN_POINT ( 'NONE',  ( 5.782158712927999211, -76.95253998579799770, 7.591266289414999591 ) ) ;
#47219=CARTESIAN_POINT ( 'NONE',  ( 5.807838419657000095, -77.18721915034599590, -7.511754867730999763 ) ) ;
#47230=VECTOR ( 'NONE', #20440, 1000.000000000000000 ) ;
#47317=CARTESIAN_POINT ( 'NONE',  ( 5.279327442448000340, -79.36243918298698929, -7.780650776298999816 ) ) ;
#47343=DIRECTION ( 'NONE',  ( 0.000000000000000000, -1.000000000000000000, 0.000000000000000000 ) ) ;
#47344=CARTESIAN_POINT ( 'NONE',  ( 0.000000000000000000, -80.79999999999999716, 0.000000000000000000 ) ) ;
#47363=CARTESIAN_POINT ( 'NONE',  ( -9.832476300866000329, -78.74688667140098630, 1.242130619674999936 ) ) ;
#47375=DIRECTION ( 'NONE',  ( 1.000000000000000000, 0.000000000000000000, 0.000000000000000000 ) ) ;
#47381=CARTESIAN_POINT ( 'NONE',  ( 2.052412689622999942, -78.08471332859899405, -9.695776403646000574 ) ) ;
#47391=ORIENTED_EDGE ( 'NONE', *, *, #24918, .F. ) ;
#47431=CARTESIAN_POINT ( 'NONE',  ( 6.174209039929378307, -79.21856170414847043, 7.219943151181964502 ) ) ;
#47436=ORIENTED_EDGE ( 'NONE', *, *, #27416, .T. ) ;
#47450=CARTESIAN_POINT ( 'NONE',  ( 0.000000000000000000, -74.70999999999999375, 0.000000000000000000 ) ) ;
#47512=DIRECTION ( 'NONE',  ( 0.000000000000000000, -1.000000000000000000, 0.000000000000000000 ) ) ;
#47548=CARTESIAN_POINT ( 'NONE',  ( 0.000000000000000000, -80.79999999999999716, 0.000000000000000000 ) ) ;
#47560=CARTESIAN_POINT ( 'NONE',  ( 9.322139347202742954, -79.52083333333069959, -1.984632903365618928 ) ) ;
#47601=( NAMED_UNIT ( * ) PLANE_ANGLE_UNIT ( ) SI_UNIT ( $, .RADIAN. ) );
#47613=CARTESIAN_POINT ( 'NONE',  ( -8.997179024602999675, -79.09910194988499654, 3.687079342327000298 ) ) ;
#47649=AXIS2_PLACEMENT_3D ( 'NONE', #2968, #56126, #16546 ) ;
#47655=CARTESIAN_POINT ( 'NONE',  ( 9.418360348373997937, -78.46536332859899687, 2.704229673158000224 ) ) ;
#47664=CARTESIAN_POINT ( 'NONE',  ( 8.002843206562671341, -77.69666666666665833, 5.305121725754474937 ) ) ;
#47676=CARTESIAN_POINT ( 'NONE',  ( -9.090572324265000503, -77.91051332859899503, 3.947417077667999763 ) ) ;
#47683=DIRECTION ( 'NONE',  ( 0.000000000000000000, -1.000000000000000000, 0.000000000000000000 ) ) ;
#47685=VERTEX_POINT ( 'NONE', #38409 ) ;
#47718=CARTESIAN_POINT ( 'NONE',  ( 3.025362517619666125, -79.24890232342751517, 9.005302098445666203 ) ) ;
#47736=EDGE_CURVE ( 'NONE', #23864, #57123, #55901, .T. ) ;
#47781=EDGE_LOOP ( 'NONE', ( #20107, #31659, #16252, #19080 ) ) ;
#47795=CARTESIAN_POINT ( 'NONE',  ( -9.648205698377651629, -78.53912913613841340, 1.218851828996400766 ) ) ;
#47801=EDGE_CURVE ( 'NONE', #18799, #36499, #57385, .T. ) ;
#47807=DIRECTION ( 'NONE',  ( -1.000000000000000000, 0.000000000000000000, 0.000000000000000000 ) ) ;
#47809=AXIS2_PLACEMENT_3D ( 'NONE', #45738, #45441, #41000 ) ;
#47839=CARTESIAN_POINT ( 'NONE',  ( 8.440830090958000298, -79.52906001420200255, -4.863879970414000553 ) ) ;
#47873=DIRECTION ( 'NONE',  ( -1.000000000000000000, 0.000000000000000000, 0.000000000000000000 ) ) ;
#47875=UNCERTAINTY_MEASURE_WITH_UNIT (LENGTH_MEASURE( 1.000000000000000082E-05 ), #376, 'distance_accuracy_value', 'NONE');
#47884=( LENGTH_UNIT ( ) NAMED_UNIT ( * ) SI_UNIT ( .MILLI., .METRE. ) );
#47895=CARTESIAN_POINT ( 'NONE',  ( -3.230363664242999810, -78.22810194988500143, -9.171071524558000121 ) ) ;
#47913=LINE ( 'NONE', #33719, #49650 ) ;
#47926=PRODUCT_DEFINITION_SHAPE ( 'NONE', 'NONE',  #4815 ) ;
#47928=ADVANCED_FACE ( 'NONE', ( #29467 ), #36786, .F. ) ;
#47943=CARTESIAN_POINT ( 'NONE',  ( 2.029274658824999911, -78.33471332859899405, -9.586470329786999756 ) ) ;
#47959=CARTESIAN_POINT ( 'NONE',  ( 6.635658238781000584, -78.32268667140098728, 7.210160158573999389 ) ) ;
#47975=CARTESIAN_POINT ( 'NONE',  ( 5.610847844242323745, -79.07500000000000284, -7.718163323371677542 ) ) ;
#48007=CARTESIAN_POINT ( 'NONE',  ( 4.262956496346735236, -79.23758755414554855, 8.489663765682541552 ) ) ;
#48040=CARTESIAN_POINT ( 'NONE',  ( 9.500000000000000000, -78.14999999999999147, 0.000000000000000000 ) ) ;
#48072=ORIENTED_EDGE ( 'NONE', *, *, #27832, .F. ) ;
#48110=ORIENTED_EDGE ( 'NONE', *, *, #3751, .T. ) ;
#48140=APPLICATION_CONTEXT ( 'automotive_design' ) ;
#48172=LINE ( 'NONE', #34553, #20619 ) ;
#48179=CARTESIAN_POINT ( 'NONE',  ( 9.500000000000000000, -78.14999999999999147, 0.000000000000000000 ) ) ;
#48182=CARTESIAN_POINT ( 'NONE',  ( -7.603664017118000551, -78.57650194988499948, 6.060370778711000384 ) ) ;
#48223=ORIENTED_EDGE ( 'NONE', *, *, #9369, .F. ) ;
#48226=CARTESIAN_POINT ( 'NONE',  ( 8.163677614451000153, -78.11386001420198966, 4.925422544966999716 ) ) ;
#48243=ORIENTED_EDGE ( 'NONE', *, *, #39099, .F. ) ;
#48266=CARTESIAN_POINT ( 'NONE',  ( 9.500000000000000000, -79.14999999999999147, 0.000000000000000000 ) ) ;
#48275=CARTESIAN_POINT ( 'NONE',  ( 5.645287065787000458, -79.33454415034599094, 7.708789581145000014 ) ) ;
#48291=CARTESIAN_POINT ( 'NONE',  ( -6.738130626923404698, -79.33754562427129997, 6.696801847776262306 ) ) ;
#48320=DIRECTION ( 'NONE',  ( 0.7071067811865474617, -0.7071067811865474617, 3.646357685208241723E-10 ) ) ;
#48356=ORIENTED_EDGE ( 'NONE', *, *, #13370, .F. ) ;
#48359=VECTOR ( 'NONE', #27747, 1000.000000000000000 ) ;
#48371=CARTESIAN_POINT ( 'NONE',  ( -7.810754875833999300, -77.80808667140099999, -5.856810041960000213 ) ) ;
#48405=CARTESIAN_POINT ( 'NONE',  ( -9.717796984206000133, -79.81506001420198970, 0.6849888841999000055 ) ) ;
#48422=ORIENTED_EDGE ( 'NONE', *, *, #13697, .F. ) ;
#48424=CARTESIAN_POINT ( 'NONE',  ( 0.000000000000000000, -75.00000000000000000, 0.000000000000000000 ) ) ;
#48459=CARTESIAN_POINT ( 'NONE',  ( -7.401612602209000968, -79.18620194988500316, -6.305503003149000030 ) ) ;
#48467=CARTESIAN_POINT ( 'NONE',  ( 0.000000000000000000, -75.20000000000000284, -11.64999999999768043 ) ) ;
#48473=CARTESIAN_POINT ( 'NONE',  ( 3.938458446976999205, -79.21000000000000796, -8.369650235310999165 ) ) ;
#48495=ORIENTED_EDGE ( 'NONE', *, *, #1134, .F. ) ;
#48500=CARTESIAN_POINT ( 'NONE',  ( -7.750101915720000179, -78.70333667140100431, 6.177086609340000756 ) ) ;
#48509=CARTESIAN_POINT ( 'NONE',  ( -8.465407715419214441, -79.43746552134066974, -4.311206955701401000 ) ) ;
#48519=CARTESIAN_POINT ( 'NONE',  ( -1.199999999999999956, -75.00000000000000000, -7.200000000000000178 ) ) ;
#48527=CARTESIAN_POINT ( 'NONE',  ( -5.838193839761688153, -78.37291666666668277, -7.596835002782716728 ) ) ;
#48551=VECTOR ( 'NONE', #17145, 1000.000000000000000 ) ;
#48562=CARTESIAN_POINT ( 'NONE',  ( 7.596835002782697188, -78.60208333333333997, 5.838193839761710358 ) ) ;
#48576=CARTESIAN_POINT ( 'NONE',  ( -1.436252226850364355, -79.28687123219287969, 9.390701153346968866 ) ) ;
#48604=CARTESIAN_POINT ( 'NONE',  ( -7.596835002782739821, -78.34791666666669130, 5.838193839761659731 ) ) ;
#48655=CARTESIAN_POINT ( 'NONE',  ( 5.073817278557999799, -78.08715333806699732, 8.075442521356999137 ) ) ;
#48687=CARTESIAN_POINT ( 'NONE',  ( -0.6048802941109999720, -79.63688667140100108, 9.614296959915000329 ) ) ;
#48707=ORIENTED_EDGE ( 'NONE', *, *, #6635, .F. ) ;
#48708=CARTESIAN_POINT ( 'NONE',  ( 7.092659876394000307, -77.99803084965400046, 6.312768414564000174 ) ) ;
#48741=CARTESIAN_POINT ( 'NONE',  ( 4.511829301271795600, -77.00000000000001421, 8.104544903090385333 ) ) ;
#48745=CARTESIAN_POINT ( 'NONE',  ( 9.377128579935000374, -78.41885584965399403, -2.571625947824999869 ) ) ;
#48757=DIRECTION ( 'NONE',  ( 0.000000000000000000, 0.000000000000000000, -1.000000000000000000 ) ) ;
#48758=CARTESIAN_POINT ( 'NONE',  ( 0.000000000000000000, -74.70999999999999375, 0.000000000000000000 ) ) ;
#48760=VECTOR ( 'NONE', #27366, 1000.000000000000000 ) ;
#48774=( NAMED_UNIT ( * ) PLANE_ANGLE_UNIT ( ) SI_UNIT ( $, .RADIAN. ) );
#48779=CARTESIAN_POINT ( 'NONE',  ( -9.500000000000001776, -78.41041666666669130, -1.243547092045959923 ) ) ;
#48806=CARTESIAN_POINT ( 'NONE',  ( -1.199999999999999956, -75.00000000000000000, 7.200000000000000178 ) ) ;
#48818=EDGE_CURVE ( 'NONE', #12545, #5875, #27040, .T. ) ;
#48845=DIRECTION ( 'NONE',  ( 0.000000000000000000, -1.000000000000000000, 0.000000000000000000 ) ) ;
#48847=EDGE_LOOP ( 'NONE', ( #14425, #27558 ) ) ;
#48856=CIRCLE ( 'NONE', #56400, 5.299999999999999822 ) ;
#48861=CARTESIAN_POINT ( 'NONE',  ( -5.443693558267039379, -79.32340947642325091, 7.785673846661049780 ) ) ;
#48867=CARTESIAN_POINT ( 'NONE',  ( 4.765028101803320482, -79.46666666666665435, -8.256991974504542142 ) ) ;
#48868=B_SPLINE_SURFACE_WITH_KNOTS ( 'NONE', 3, 3, ( 
 ( #6260, #47317, #19269, #24275, #42293, #41700, #1858, #14820, #19853, #37848, #47027, #6557, #24565, #20147, #38134, #39294, #44304, #43164, #7427, #52310, #26291, #3860, #29843, #48745, #11579, #8288, #57587, #53166, #25430, #16869, #7137, #52595, #21858, #30708, #29558 ),
 ( #43445, #21002, #16578, #39867, #48459, #57306, #47613, #57880, #39583, #30133, #34848, #17437, #17148, #16298, #35135, #12715, #52880, #35422, #48182, #25138, #34275, #20717, #2721, #38717, #11866, #56738, #47895, #3006, #25999, #39008, #57016, #34563, #12146, #7715, #25716 ),
 ( #12434, #43742, #30427, #3295, #21287, #8002, #44022, #3574, #21579, #31877, #49921, #10563, #9466, #49328, #27451, #22152, #31580, #42144, #54343, #6121, #348, #4448, #26868, #44599, #13883, #58173, #51013, #24126, #22449, #46595, #4153, #40464, #17739, #49626, #45489 ),
 ( #40160, #28546, #19706, #1713, #53452, #22744, #5032, #9173, #23034, #41050, #40754, #18327, #35727, #55426, #1426, #19415, #13291, #37405, #26567, #36320, #56, #14972, #53754, #27156, #12997, #32969, #30994, #49032, #18031, #44896, #31285, #8580, #8874, #36023, #54050 ) ),
 .UNSPECIFIED., .F., .F., .F.,
 ( 4, 4 ),
 ( 4, 1, 1, 1, 1, 1, 1, 1, 1, 1, 1, 1, 1, 1, 1, 1, 1, 1, 1, 1, 1, 1, 1, 1, 1, 1, 1, 1, 1, 1, 1, 1, 4 ),
 ( -0.4015584965371999937, 1.401558496537000043 ),
 ( -0.02000000000000000042, 0.01250000000000000069, 0.04499999999999999833, 0.07749999999999999944, 0.1100000000000000006, 0.1424999999999999878, 0.1749999999999999889, 0.2074999999999999900, 0.2399999999999999911, 0.2725000000000000200, 0.3049999999999999933, 0.3375000000000000222, 0.3699999999999999956, 0.4025000000000000244, 0.4349999999999999978, 0.4675000000000000266, 0.5000000000000000000, 0.5324999999999999734, 0.5649999999999999467, 0.5975000000000000311, 0.6300000000000000044, 0.6624999999999999778, 0.6949999999999999512, 0.7275000000000000355, 0.7600000000000000089, 0.7924999999999999822, 0.8249999999999999556, 0.8575000000000000400, 0.8900000000000000133, 0.9224999999999999867, 0.9549999999999999600, 0.9875000000000000444, 1.020000000000000018 ),
 .UNSPECIFIED. ) ;
#48871=ADVANCED_FACE ( 'NONE', ( #845 ), #23250, .T. ) ;
#48884=DIRECTION ( 'NONE',  ( 0.000000000000000000, 0.000000000000000000, -1.000000000000000000 ) ) ;
#48892=B_SPLINE_CURVE_WITH_KNOTS ( 'NONE', 3,
 ( #48473, #51756, #20737, #2448 ),
 .UNSPECIFIED., .F., .F.,
 ( 4, 4 ),
 ( 0.000000000000000000, 1.000000000000000000 ),
 .UNSPECIFIED. ) ;
#48898=CARTESIAN_POINT ( 'NONE',  ( 8.119885838724000493, -79.78146001420199696, -4.358224697923000157 ) ) ;
#48922=AXIS2_PLACEMENT_3D ( 'NONE', #38632, #11778, #47807 ) ;
#48933=CARTESIAN_POINT ( 'NONE',  ( 1.229229938689273993, -79.60286458332932114, 9.397135416583925149 ) ) ;
#48940=CARTESIAN_POINT ( 'NONE',  ( 8.241485672608000357, -77.61706001420199641, 5.435909736561999495 ) ) ;
#48995=CARTESIAN_POINT ( 'NONE',  ( 8.503129636637000388, -77.90345584965399439, -4.225430575863000193 ) ) ;
#49018=CARTESIAN_POINT ( 'NONE',  ( 8.914106061823998672, -77.72396332859899815, 3.639947156824000274 ) ) ;
#49032=CARTESIAN_POINT ( 'NONE',  ( -7.530775182571000315, -78.06434415034598828, -6.150709233331999037 ) ) ;
#49038=CARTESIAN_POINT ( 'NONE',  ( -5.610847844242281113, -78.22500000000000853, 7.718163323371710405 ) ) ;
#49066=CARTESIAN_POINT ( 'NONE',  ( 5.838193839761703252, -78.57708333333333428, -7.596835002782702517 ) ) ;
#49067=CARTESIAN_POINT ( 'NONE',  ( 9.254623623301998947, -77.89893998579799472, 2.326634063882999648 ) ) ;
#49083=CARTESIAN_POINT ( 'NONE',  ( -6.047833114999293436, -79.47011274197635089, -7.345927578306194583 ) ) ;
#49085=CARTESIAN_POINT ( 'NONE',  ( 0.9993909113990739890, -79.43417149341397021, -9.481187304795884785 ) ) ;
#49093=CIRCLE ( 'NONE', #53818, 11.65000000000000036 ) ;
#49127=DIRECTION ( 'NONE',  ( 1.000000000000000000, 0.000000000000000000, 0.000000000000000000 ) ) ;
#49142=ADVANCED_FACE ( 'NONE', ( #9961 ), #25750, .T. ) ;
#49149=CARTESIAN_POINT ( 'NONE',  ( -0.1688430469021683922, -79.27612716086017031, 9.502712028091975682 ) ) ;
#49162=CARTESIAN_POINT ( 'NONE',  ( 8.745915541949560890, -77.83069693750340434, 3.571268974134527152 ) ) ;
#49181=EDGE_CURVE ( 'NONE', #10450, #22499, #42753, .T. ) ;
#49184=CARTESIAN_POINT ( 'NONE',  ( -6.137787596906999710, -79.43688667140099824, 7.419310695580000115 ) ) ;
#49222=CIRCLE ( 'NONE', #18929, 9.199999999999999289 ) ;
#49225=CARTESIAN_POINT ( 'NONE',  ( 2.460597061978947675, -79.59635416666264973, 9.159220229803393565 ) ) ;
#49232=CARTESIAN_POINT ( 'NONE',  ( 0.7109233471628000345, -77.62608667140099783, 9.736770704497999418 ) ) ;
#49268=CARTESIAN_POINT ( 'NONE',  ( 9.505044359491998662, -79.49388667140100040, -1.566734738709000041 ) ) ;
#49291=CARTESIAN_POINT ( 'NONE',  ( 8.256620083228000340, -77.39905584965399044, -4.688888258373000717 ) ) ;
#49312=CARTESIAN_POINT ( 'NONE',  ( 7.497416719750999548, -77.63913832859898889, -6.041447127439999676 ) ) ;
#49328=CARTESIAN_POINT ( 'NONE',  ( 4.598371993787000456, -78.73414805011499595, -8.567308531191999421 ) ) ;
#49337=CARTESIAN_POINT ( 'NONE',  ( 4.594620150137029846, -78.13500000000000512, 8.363081028749705936 ) ) ;
#49349=FACE_BOUND ( 'NONE', #30248, .T. ) ;
#49363=CARTESIAN_POINT ( 'NONE',  ( -7.596835002782708735, -78.45208333333333428, -5.838193839761694370 ) ) ;
#49384=CARTESIAN_POINT ( 'NONE',  ( -8.466964544433025708, -79.43743728541620897, -4.308145801908138672 ) ) ;
#49387=DIRECTION ( 'NONE',  ( 0.000000000000000000, -1.000000000000000000, 0.000000000000000000 ) ) ;
#49454=CARTESIAN_POINT ( 'NONE',  ( -4.760392715106998907, -79.31640648056026066, 8.226848814529617471 ) ) ;
#49499=ORIENTED_EDGE ( 'NONE', *, *, #8298, .F. ) ;
#49504=ORIENTED_EDGE ( 'NONE', *, *, #32734, .F. ) ;
#49507=CARTESIAN_POINT ( 'NONE',  ( 0.000000000000000000, -75.10000000019110189, 0.000000000000000000 ) ) ;
#49512=ORIENTED_EDGE ( 'NONE', *, *, #23501, .F. ) ;
#49518=ADVANCED_FACE ( 'NONE', ( #23313 ), #34242, .T. ) ;
#49536=CARTESIAN_POINT ( 'NONE',  ( -9.851679666438998950, -77.32586001420199295, -0.6446771120444999559 ) ) ;
#49574=CARTESIAN_POINT ( 'NONE',  ( -1.884618100832999854, -79.80191332859899944, -9.129359532056000148 ) ) ;
#49594=VERTEX_POINT ( 'NONE', #9975 ) ;
#49595=CARTESIAN_POINT ( 'NONE',  ( 9.426477049435000310, -77.31037305011500393, -1.139727483088999849 ) ) ;
#49615=CARTESIAN_POINT ( 'NONE',  ( -7.080509631177999808, -76.88513832859899821, 6.324808343700000002 ) ) ;
#49625=DIRECTION ( 'NONE',  ( 0.8090169943750002979, 0.000000000000000000, -0.5877852522924001955 ) ) ;
#49626=CARTESIAN_POINT ( 'NONE',  ( 7.048436826466999428, -77.87766471678199309, 6.223291978577000449 ) ) ;
#49650=VECTOR ( 'NONE', #11597, 1000.000000000000000 ) ;
#49659=CARTESIAN_POINT ( 'NONE',  ( 9.500000000000001776, -78.63958333333336270, -1.243547092045940827 ) ) ;
#49660=CARTESIAN_POINT ( 'NONE',  ( 5.722682530001000245, -76.87071332859899542, -7.358525362622999388 ) ) ;
#49664=EDGE_LOOP ( 'NONE', ( #29029, #3618, #54745, #35679, #37865 ) ) ;
#49673=CARTESIAN_POINT ( 'NONE',  ( 11.44999999995999929, -74.99999999996168754, 1.667679908953999909E-09 ) ) ;
#49681=CARTESIAN_POINT ( 'NONE',  ( -8.499390037608824500, -79.43684124743761288, -4.243882634569263068 ) ) ;
#49713=CARTESIAN_POINT ( 'NONE',  ( 5.896171905175000560, -77.86999999999999034, 7.127247495676000355 ) ) ;
#49749=CARTESIAN_POINT ( 'NONE',  ( -7.699832853999788895, -79.34979350599515158, 5.563995025944507233 ) ) ;
#49750=CARTESIAN_POINT ( 'NONE',  ( 11.44999999999999929, -75.00000000000000000, 0.000000000000000000 ) ) ;
#49754=ORIENTED_EDGE ( 'NONE', *, *, #58236, .T. ) ;
#49783=CARTESIAN_POINT ( 'NONE',  ( 2.759513673833999814, -79.21986001420199841, -8.792710209907999896 ) ) ;
#49788=ADVANCED_FACE ( 'NONE', ( #42000 ), #1568, .F. ) ;
#49805=ORIENTED_EDGE ( 'NONE', *, *, #29182, .F. ) ;
#49808=VERTEX_POINT ( 'NONE', #39014 ) ;
#49832=DIRECTION ( 'NONE',  ( 0.000000000000000000, 0.000000000000000000, -1.000000000000000000 ) ) ;
#49835=CARTESIAN_POINT ( 'NONE',  ( -2.935661446561999899, -77.00000000000000000, -9.035036904803998681 ) ) ;
#49870=CARTESIAN_POINT ( 'NONE',  ( -5.025355631522999467, -79.70953998579798849, -7.962943362895000377 ) ) ;
#49889=CARTESIAN_POINT ( 'NONE',  ( -6.013262726775999489, -77.49952305011500187, 7.348341287529000176 ) ) ;
#49908=CARTESIAN_POINT ( 'NONE',  ( 2.191831765174000246, -77.29983832859899451, 9.375831637944999741 ) ) ;
#49913=EDGE_CURVE ( 'NONE', #13828, #31238, #39648, .T. ) ;
#49918=CARTESIAN_POINT ( 'NONE',  ( 9.267587667790845529, -76.99999999999998579, 1.705438069304222370 ) ) ;
#49921=CARTESIAN_POINT ( 'NONE',  ( 8.219513559211000242, -78.86479805011499877, 5.194554602171000290 ) ) ;
#49926=EDGE_LOOP ( 'NONE', ( #10585, #5787, #18049 ) ) ;
#49946=EDGE_CURVE ( 'NONE', #39734, #44850, #2438, .T. ) ;
#49949=SURFACE_STYLE_USAGE ( .BOTH. , #45520 ) ;
#49977=DIRECTION ( 'NONE',  ( 1.000000000000000000, 0.000000000000000000, 0.000000000000000000 ) ) ;
#50000=CARTESIAN_POINT ( 'NONE',  ( 8.503129636637000388, -77.86329903538302233, -4.225430575863000193 ) ) ;
#50006=CARTESIAN_POINT ( 'NONE',  ( 1.452949461559788435, -79.75000000000001421, -9.164018243494927773 ) ) ;
#50020=EDGE_CURVE ( 'NONE', #24677, #31756, #14287, .T. ) ;
#50076=CARTESIAN_POINT ( 'NONE',  ( -2.382925498960999811, -79.40178667140099833, 9.329537718716998995 ) ) ;
#50093=VERTEX_POINT ( 'NONE', #31478 ) ;
#50097=DIRECTION ( 'NONE',  ( 0.000000000000000000, 1.000000000000000000, 0.000000000000000000 ) ) ;
#50105=CARTESIAN_POINT ( 'NONE',  ( 9.383705654690636777, -79.16227050890121575, 1.484107674336303972 ) ) ;
#50108=B_SPLINE_CURVE_WITH_KNOTS ( 'NONE', 3,
 ( #5843, #45733, #6137, #18852, #27401, #50446, #22985, #5268, #23277, #41282, #866, #32402, #10880 ),
 .UNSPECIFIED., .F., .F.,
 ( 4, 1, 2, 2, 2, 2, 4 ),
 ( 0.000000000000000000, 0.1250000000000001110, 0.1875000000000000833, 0.2500000000000000555, 0.5000000000000000000, 0.7500000000000000000, 1.000000000000000000 ),
 .UNSPECIFIED. ) ;
#50120=FACE_OUTER_BOUND ( 'NONE', #57841, .T. ) ;
#50121=DIRECTION ( 'NONE',  ( 0.000000000000000000, 1.000000000000000000, 0.000000000000000000 ) ) ;
#50127=CARTESIAN_POINT ( 'NONE',  ( -5.375314035255999379, -77.27111332859900017, -8.017434526278000462 ) ) ;
#50141=DIRECTION ( 'NONE',  ( 0.000000000000000000, 1.000000000000000000, -4.736951571734000187E-14 ) ) ;
#50160=CARTESIAN_POINT ( 'NONE',  ( 5.983750641729000286, -79.30913998579799795, -7.270309104952999313 ) ) ;
#50179=CARTESIAN_POINT ( 'NONE',  ( -5.597970637881999778, -76.99512305011499791, 7.669424558767000022 ) ) ;
#50187=CARTESIAN_POINT ( 'NONE',  ( 4.784380313523521444, -77.63333333333332575, 8.300970689365463784 ) ) ;
#50194=DIRECTION ( 'NONE',  ( -1.000000000000000000, 0.000000000000000000, 0.000000000000000000 ) ) ;
#50195=CARTESIAN_POINT ( 'NONE',  ( -2.745946062086999984, -76.98158998579799572, -9.341962526838999636 ) ) ;
#50219=CARTESIAN_POINT ( 'NONE',  ( 0.000000000000000000, -75.00000000000000000, -11.45000000000000107 ) ) ;
#50230=B_SPLINE_CURVE_WITH_KNOTS ( 'NONE', 3,
 ( #7711, #44019, #3571, #35131, #53163, #2717, #30705, #57013, #48741, #8285, #17434, #20714, #27153, #23329, #13289, #17736, #26564, #32165, #8872, #45786, #36895, #44894, #18618, #41336, #8577, #4445, #4742, #32452, #9464, #49918, #636, #27449, #18325, #41047, #44595, #346, #9171, #14167, #5321 ),
 .UNSPECIFIED., .F., .F.,
 ( 4, 1, 1, 1, 1, 1, 2, 2, 1, 1, 1, 1, 2, 2, 1, 1, 2, 2, 2, 2, 2, 2, 2, 2, 4 ),
 ( 0.000000000000000000, 0.06249999999999412970, 0.09374999999999117373, 0.1093749999999896888, 0.1171874999999888700, 0.1210937499999883704, 0.1230468749999882871, 0.1249999999999882039, 0.1874999999999883149, 0.2187499999999883982, 0.2343749999999884259, 0.2421874999999883704, 0.2460937499999883427, 0.2499999999999883427, 0.3124999999999890643, 0.3437499999999893419, 0.3593749999999896194, 0.3749999999999898415, 0.4374999999999908407, 0.4999999999999918954, 0.6249999999999938938, 0.7499999999999958922, 0.8124999999999970024, 0.8749999999999980016, 1.000000000000000000 ),
 .UNSPECIFIED. ) ;
#50240=CARTESIAN_POINT ( 'NONE',  ( -3.329695900066999670, -77.97738998579799841, -9.453077866293002174 ) ) ;
#50297=DIRECTION ( 'NONE',  ( -1.000000000000000000, 0.000000000000000000, 0.000000000000000000 ) ) ;
#50318=ORIENTED_EDGE ( 'NONE', *, *, #16182, .F. ) ;
#50345=CARTESIAN_POINT ( 'NONE',  ( 8.283364115789000337, -78.80173667140100235, 5.234906771447999319 ) ) ;
#50376=CARTESIAN_POINT ( 'NONE',  ( 9.539544502573999551, -79.38455194988500807, 0.5400218831817999998 ) ) ;
#50377=DIRECTION ( 'NONE',  ( 0.000000000000000000, 0.000000000000000000, -1.000000000000000000 ) ) ;
#50389=ORIENTED_EDGE ( 'NONE', *, *, #25804, .T. ) ;
#50410=CARTESIAN_POINT ( 'NONE',  ( 7.011029437969999556, -77.81601167140100017, 6.440258933668999930 ) ) ;
#50446=CARTESIAN_POINT ( 'NONE',  ( -5.624774363530229415, -76.99999999999998579, 7.347433795508993448 ) ) ;
#50450=CARTESIAN_POINT ( 'NONE',  ( 9.290732676231000298, -79.36633998579799254, -1.531409331864000078 ) ) ;
#50455=CONICAL_SURFACE ( 'NONE', #43834, 9.334374999970000530, 0.7853981633972997312 ) ;
#50471=CARTESIAN_POINT ( 'NONE',  ( -7.264520526674999701, -77.68572694988499450, -6.114261184555999762 ) ) ;
#50496=LINE ( 'NONE', #28032, #9797 ) ;
#50523=CARTESIAN_POINT ( 'NONE',  ( -9.330562018306766348, -76.99999999999997158, -0.3894759657577204215 ) ) ;
#50531=ORIENTED_EDGE ( 'NONE', *, *, #48818, .F. ) ;
#50532=CARTESIAN_POINT ( 'NONE',  ( -5.941820572504999731, -78.80483998579799731, 8.071079272148001138 ) ) ;
#50545=FACE_OUTER_BOUND ( 'NONE', #52898, .T. ) ;
#50619=CARTESIAN_POINT ( 'NONE',  ( 6.682297893293000612, -79.50746001420199605, -6.800905403285999462 ) ) ;
#50642=FACE_OUTER_BOUND ( 'NONE', #18866, .T. ) ;
#50658=CARTESIAN_POINT ( 'NONE',  ( 5.754008857420999767, -79.26781332859900431, 7.857252078236999004 ) ) ;
#50670=CARTESIAN_POINT ( 'NONE',  ( -8.650571159592999493, -79.59515194988499331, 4.057379972786000266 ) ) ;
#50671=DIRECTION ( 'NONE',  ( 0.000000000000000000, 1.000000000000000000, 0.000000000000000000 ) ) ;
#50673=AXIS2_PLACEMENT_3D ( 'NONE', #39140, #43877, #52727 ) ;
#50679=LINE ( 'NONE', #23788, #10491 ) ;
#50693=ORIENTED_EDGE ( 'NONE', *, *, #42170, .F. ) ;
#50703=ADVANCED_FACE ( 'NONE', ( #227 ), #26479, .F. ) ;
#50704=CARTESIAN_POINT ( 'NONE',  ( 0.000000000000000000, -76.00000000000000000, 0.000000000000000000 ) ) ;
#50707=CARTESIAN_POINT ( 'NONE',  ( 7.328371322744000160, -77.76668501420199675, -5.905229698647000092 ) ) ;
#50713=FACE_OUTER_BOUND ( 'NONE', #25941, .T. ) ;
#50716=CARTESIAN_POINT ( 'NONE',  ( 2.946159983835261897, -77.05000000000001137, -9.062386480552282464 ) ) ;
#50744=EDGE_LOOP ( 'NONE', ( #17484, #19228, #21650, #8914 ) ) ;
#50767=CARTESIAN_POINT ( 'NONE',  ( -8.123853732960998997, -77.08675194988499868, 4.915330883505999893 ) ) ;
#50780=ADVANCED_FACE ( 'NONE', ( #55079 ), #4241, .F. ) ;
#50791=CARTESIAN_POINT ( 'NONE',  ( 0.000000000000000000, -75.10000000284179578, -8.299999997157998521 ) ) ;
#50818=CARTESIAN_POINT ( 'NONE',  ( -7.034477742621340290, -76.99999999999998579, -6.292097733782652469 ) ) ;
#50825=CARTESIAN_POINT ( 'NONE',  ( 4.594620150137028958, -77.73500000000001364, 8.363081028749707713 ) ) ;
#50832=CARTESIAN_POINT ( 'NONE',  ( -7.664471376495262334, -79.34928386457644933, 5.612613647751031110 ) ) ;
#50838=DIRECTION ( 'NONE',  ( 0.000000000000000000, -1.000000000000000000, 0.000000000000000000 ) ) ;
#50854=CARTESIAN_POINT ( 'NONE',  ( 7.553659961756574504, -79.10220767479606252, 5.794321821515795889 ) ) ;
#50915=CARTESIAN_POINT ( 'NONE',  ( 9.188870790291835178, -77.67333333333333201, 2.784684813981615825 ) ) ;
#50929=CARTESIAN_POINT ( 'NONE',  ( 4.299985066278999568, -78.90906001420199800, 8.680515821880000260 ) ) ;
#50952=CARTESIAN_POINT ( 'NONE',  ( 4.598371993787000456, -78.81419514476064592, -8.567308531191999421 ) ) ;
#50955=CARTESIAN_POINT ( 'NONE',  ( -8.650571159592999493, -79.53504805011499457, 4.057379972786000266 ) ) ;
#50956=CARTESIAN_POINT ( 'NONE',  ( 0.000000000000000000, -80.79999999999999716, -6.099999999999782041 ) ) ;
#50960=CARTESIAN_POINT ( 'NONE',  ( 7.069026043852319141, -79.73437500013776003, -6.033943149941224604 ) ) ;
#50996=CARTESIAN_POINT ( 'NONE',  ( 4.194094809819000069, -77.90806001420200744, 8.205866028503001175 ) ) ;
#51002=CARTESIAN_POINT ( 'NONE',  ( -9.486170818179999742, -77.70791332859900535, -1.784886728388999977 ) ) ;
#51013=CARTESIAN_POINT ( 'NONE',  ( -3.230363664242999810, -78.16799805011500268, -9.171071524558000121 ) ) ;
#51075=CARTESIAN_POINT ( 'NONE',  ( 6.055527902613000002, -78.11999999999999034, 7.319875806370000682 ) ) ;
#51079=ORIENTED_EDGE ( 'NONE', *, *, #29959, .F. ) ;
#51121=CARTESIAN_POINT ( 'NONE',  ( -0.5475862000146000108, -78.49998998579799547, -10.00738244094000073 ) ) ;
#51144=CARTESIAN_POINT ( 'NONE',  ( -9.292748675297000105, -77.02431167140100854, -2.067979918156000352 ) ) ;
#51146=CARTESIAN_POINT ( 'NONE',  ( 8.244744731391815407, -79.09176881386157731, 4.761212502374692512 ) ) ;
#51167=DIRECTION ( 'NONE',  ( 1.000000000000000000, 0.000000000000000000, 0.000000000000000000 ) ) ;
#51224=CARTESIAN_POINT ( 'NONE',  ( 8.188916213828999702, -78.86551001420200180, 5.175217742376999830 ) ) ;
#51272=CARTESIAN_POINT ( 'NONE',  ( 9.035652705983848065, -79.17456789375879112, 2.932964697886948802 ) ) ;
#51289=CARTESIAN_POINT ( 'NONE',  ( 4.816281158205000246, -77.73841001420198893, -8.085802691758997796 ) ) ;
#51304=CARTESIAN_POINT ( 'NONE',  ( 3.938458446976999205, -79.30999999999998806, -8.369650235310999165 ) ) ;
#51311=VERTEX_POINT ( 'NONE', #36565 ) ;
#51314=ADVANCED_FACE ( 'NONE', ( #13834 ), #39606, .F. ) ;
#51336=EDGE_LOOP ( 'NONE', ( #48243, #1540, #22186, #742, #19965, #35164, #19581 ) ) ;
#51340=EDGE_LOOP ( 'NONE', ( #19859, #47436, #49504, #34092 ) ) ;
#51345=CARTESIAN_POINT ( 'NONE',  ( -8.383077572658999443, -77.47094415034599990, 4.458862939031999595 ) ) ;
#51349=CARTESIAN_POINT ( 'NONE',  ( 9.378599967755729239, -78.27782913613843618, -2.572029467843342854 ) ) ;
#51411=CARTESIAN_POINT ( 'NONE',  ( 4.634228027295999475, -77.71608998579800698, 8.886345528036001085 ) ) ;
#51416=CARTESIAN_POINT ( 'NONE',  ( -9.465687769217371539, -79.39306401481779574, 0.8068586129222159453 ) ) ;
#51512=CARTESIAN_POINT ( 'NONE',  ( -7.750101915720000179, -78.38956332859899589, 6.177086609340000756 ) ) ;
#51519=FACE_OUTER_BOUND ( 'NONE', #2315, .T. ) ;
#51535=CARTESIAN_POINT ( 'NONE',  ( -9.738811118029000014, -79.44331332859900385, -0.02447652147661999802 ) ) ;
#51539=CARTESIAN_POINT ( 'NONE',  ( -0.8481231068849000021, -79.03194514476065535, 9.686304223355000076 ) ) ;
#51543=CARTESIAN_POINT ( 'NONE',  ( 7.507056363060000237, -79.88925584965399196, -5.572808305725000189 ) ) ;
#51548=CARTESIAN_POINT ( 'NONE',  ( -9.500000000000000000, -77.38958333333332007, 1.243547092045920399 ) ) ;
#51562=CARTESIAN_POINT ( 'NONE',  ( 4.313834340563736269, -79.23712179264661870, 8.463837022421156320 ) ) ;
#51585=CARTESIAN_POINT ( 'NONE',  ( 7.596835002782697188, -77.10208333333333997, 5.838193839761710358 ) ) ;
#51613=AXIS2_PLACEMENT_3D ( 'NONE', #35826, #45295, #49127 ) ;
#51617=ADVANCED_FACE ( 'NONE', ( #23212 ), #12431, .F. ) ;
#51634=CARTESIAN_POINT ( 'NONE',  ( -5.314024065878000691, -77.20733998579800073, -7.926018785099000041 ) ) ;
#51641=CARTESIAN_POINT ( 'NONE',  ( 9.475051992780000987, -77.75466915034600390, -0.6170397550469999270 ) ) ;
#51656=CARTESIAN_POINT ( 'NONE',  ( -9.500000000000000000, -77.89999999999999147, 0.000000000000000000 ) ) ;
#51661=CARTESIAN_POINT ( 'NONE',  ( 5.838193839761669501, -78.72291666666666288, 7.596835002782726498 ) ) ;
#51693=CARTESIAN_POINT ( 'NONE',  ( -8.627274293348017764, -77.00000000000002842, 3.431425210218347122 ) ) ;
#51747=DIRECTION ( 'NONE',  ( 0.000000000000000000, 1.000000000000000000, 0.000000000000000000 ) ) ;
#51756=CARTESIAN_POINT ( 'NONE',  ( 3.973865631610368432, -79.15970006417956029, -8.444888605590360697 ) ) ;
#51771=B_SPLINE_CURVE_WITH_KNOTS ( 'NONE', 3,
 ( #37972, #11994, #6976, #25556 ),
 .UNSPECIFIED., .F., .F.,
 ( 4, 4 ),
 ( 0.7499999933975610711, 1.000000000000000000 ),
 .UNSPECIFIED. ) ;
#51786=CARTESIAN_POINT ( 'NONE',  ( 9.797588846018999931, -78.94441332859899774, 0.1600704101387999956 ) ) ;
#51802=CARTESIAN_POINT ( 'NONE',  ( -0.8644569908188000085, -78.82506332859900056, 9.872851397518997985 ) ) ;
#51811=DIRECTION ( 'NONE',  ( 0.000000000000000000, -1.000000000000000000, 0.000000000000000000 ) ) ;
#51814=CARTESIAN_POINT ( 'NONE',  ( -9.500000000000000000, -77.39999999999999147, 0.000000000000000000 ) ) ;
#51825=DIRECTION ( 'NONE',  ( 0.000000000000000000, 1.000000000000000000, 0.000000000000000000 ) ) ;
#51831=DIRECTION ( 'NONE',  ( 0.000000000000000000, 1.000000000000000000, 0.000000000000000000 ) ) ;
#51848=CARTESIAN_POINT ( 'NONE',  ( 7.698542609049095375, -79.19952453424221517, 5.565885376627822900 ) ) ;
#51867=CARTESIAN_POINT ( 'NONE',  ( -1.193181427976999887, -77.39188667140099653, 9.445003550666001502 ) ) ;
#51870=CARTESIAN_POINT ( 'NONE',  ( 8.300970689365438915, -77.09166666666668277, 4.784380313523563188 ) ) ;
#51879=CARTESIAN_POINT ( 'NONE',  ( -4.784380313523575623, -78.31666666666669130, 8.300970689365433586 ) ) ;
#51915=( GEOMETRIC_REPRESENTATION_CONTEXT ( 3 ) GLOBAL_UNCERTAINTY_ASSIGNED_CONTEXT ( ( #47875 ) ) GLOBAL_UNIT_ASSIGNED_CONTEXT ( ( #376, #48774, #4186 ) ) REPRESENTATION_CONTEXT ( 'NONE', 'WORKASPACE' ) );
#51916=CARTESIAN_POINT ( 'NONE',  ( 9.542482966934999311, -76.87973998579799684, 0.04799272824659999576 ) ) ;
#51922=AXIS2_PLACEMENT_3D ( 'NONE', #52619, #47343, #43766 ) ;
#51925=CARTESIAN_POINT ( 'NONE',  ( -0.7479529023060000892, -77.62856915034599581, -9.465622776916999825 ) ) ;
#51929=CARTESIAN_POINT ( 'NONE',  ( 5.896171905175000560, -77.86999999999999034, 7.127247495676000355 ) ) ;
#51935=EDGE_CURVE ( 'NONE', #10344, #8584, #37364, .T. ) ;
#51942=CARTESIAN_POINT ( 'NONE',  ( -9.500000000000000000, -78.88958333333330586, 1.243547092045920399 ) ) ;
#51971=CARTESIAN_POINT ( 'NONE',  ( 7.685661446562000343, -79.50000000000000000, -5.583959896778000420 ) ) ;
#52006=UNCERTAINTY_MEASURE_WITH_UNIT (LENGTH_MEASURE( 1.000000000000000082E-05 ), #38750, 'distance_accuracy_value', 'NONE');
#52026=DIRECTION ( 'NONE',  ( -8.742284675758000260E-11, -1.000000000000000000, -2.562965951460999736E-09 ) ) ;
#52064=ORIENTED_EDGE ( 'NONE', *, *, #3816, .F. ) ;
#52069=CARTESIAN_POINT ( 'NONE',  ( 1.914689014128999833, -78.55246332859900349, 9.610012265935001352 ) ) ;
#52071=FACE_OUTER_BOUND ( 'NONE', #45480, .T. ) ;
#52073=ORIENTED_EDGE ( 'NONE', *, *, #23431, .T. ) ;
#52086=CARTESIAN_POINT ( 'NONE',  ( 7.981661899572999985, -77.80008667140099021, 4.815606314103999530 ) ) ;
#52100=CARTESIAN_POINT ( 'NONE',  ( 7.685661446562000343, -79.50000000000000000, -5.583959896778000420 ) ) ;
#52109=FACE_BOUND ( 'NONE', #49926, .T. ) ;
#52113=CARTESIAN_POINT ( 'NONE',  ( -7.401612602209000968, -79.20614514476065438, -6.305503003149000030 ) ) ;
#52124=CARTESIAN_POINT ( 'NONE',  ( 4.784380313523521444, -78.63333333333332575, 8.300970689365463784 ) ) ;
#52127=ADVANCED_FACE ( 'NONE', ( #33517 ), #30813, .T. ) ;
#52135=CARTESIAN_POINT ( 'NONE',  ( 4.159563559845795844, -79.23853427882175993, 8.541212464559901463 ) ) ;
#52146=EDGE_CURVE ( 'NONE', #22854, #2820, #49222, .T. ) ;
#52154=CARTESIAN_POINT ( 'NONE',  ( 1.722150539371000155, -77.64636167140099587, -9.363010803921000047 ) ) ;
#52191=AXIS2_PLACEMENT_3D ( 'NONE', #55709, #6104, #45402 ) ;
#52199=CONICAL_SURFACE ( 'NONE', #19079, 5.199999999809000073, 0.7853981633972997312 ) ;
#52206=CARTESIAN_POINT ( 'NONE',  ( 4.897371265365999982, -76.90054805011499184, 7.847181321287999722 ) ) ;
#52211=CARTESIAN_POINT ( 'NONE',  ( 5.896171905175000560, -77.96999999999999886, 7.127247495676000355 ) ) ;
#52217=CARTESIAN_POINT ( 'NONE',  ( -7.471200359486886988, -79.35399621689622052, -5.924110288814695480 ) ) ;
#52222=CARTESIAN_POINT ( 'NONE',  ( -9.500000000000000000, -78.89999999999999147, 0.000000000000000000 ) ) ;
#52238=ORIENTED_EDGE ( 'NONE', *, *, #20894, .F. ) ;
#52258=CARTESIAN_POINT ( 'NONE',  ( -7.880615083743071736, -76.99999999999998579, 4.906469375586612003 ) ) ;
#52263=AXIS2_PLACEMENT_3D ( 'NONE', #54794, #14336, #28195 ) ;
#52272=CARTESIAN_POINT ( 'NONE',  ( -2.935661446561999899, -79.50000000000000000, -9.035036904803998681 ) ) ;
#52288=CARTESIAN_POINT ( 'NONE',  ( 0.000000000000000000, -78.00000000000000000, 7.200000000000000178 ) ) ;
#52301=EDGE_CURVE ( 'NONE', #15146, #34611, #49093, .T. ) ;
#52310=CARTESIAN_POINT ( 'NONE',  ( -3.339615680726000235, -78.59305584965399305, 9.131854552393999569 ) ) ;
#52355=CARTESIAN_POINT ( 'NONE',  ( 6.721258625739999992, -78.37826332859900447, -7.130431436203999773 ) ) ;
#52374=CARTESIAN_POINT ( 'NONE',  ( 8.377812017747999107, -78.73796332859900815, 5.294595800518999695 ) ) ;
#52396=CARTESIAN_POINT ( 'NONE',  ( 0.000000000000000000, -75.00000000000000000, 0.000000000000000000 ) ) ;
#52397=PLANE ( 'NONE',  #33489 ) ;
#52410=CARTESIAN_POINT ( 'NONE',  ( -9.500000000000007105, -78.78958333333333997, 1.243547092045919733 ) ) ;
#52411=DIRECTION ( 'NONE',  ( -1.000000000000000000, 0.000000000000000000, 0.000000000000000000 ) ) ;
#52420=CARTESIAN_POINT ( 'NONE',  ( 2.753209777146519599, -79.25137801636039114, 9.093106921346176819 ) ) ;
#52452=ADVANCED_FACE ( 'NONE', ( #7731 ), #55723, .F. ) ;
#52471=DIRECTION ( 'NONE',  ( 0.8090169943749183634, 0.000000000000000000, -0.5877852522925132162 ) ) ;
#52472=CIRCLE ( 'NONE', #1581, 11.65000000000000036 ) ;
#52494=CARTESIAN_POINT ( 'NONE',  ( -3.230870548382956287, -78.14717913613844757, -9.172510579469401293 ) ) ;
#52501=CARTESIAN_POINT ( 'NONE',  ( 7.747477005942000616, -78.01746001420200116, -6.119465872965999864 ) ) ;
#52505=CARTESIAN_POINT ( 'NONE',  ( -2.486604901413195901, -78.79583333333337691, 9.252740428348989354 ) ) ;
#52506=AXIS2_PLACEMENT_3D ( 'NONE', #30776, #53522, #26352 ) ;
#52531=ORIENTED_EDGE ( 'NONE', *, *, #55086, .F. ) ;
#52534=CARTESIAN_POINT ( 'NONE',  ( -9.609463960252000447, -79.75128667140099026, 0.6773526969735000902 ) ) ;
#52539=VERTEX_POINT ( 'NONE', #36625 ) ;
#52541=CARTESIAN_POINT ( 'NONE',  ( -8.749250031325688681, -76.99999999999998579, 3.121704046829004486 ) ) ;
#52555=CARTESIAN_POINT ( 'NONE',  ( 5.102724688570000389, -77.95894361655099658, 7.811319209985999379 ) ) ;
#52557=AXIS2_PLACEMENT_3D ( 'NONE', #42117, #55103, #5797 ) ;
#52582=CARTESIAN_POINT ( 'NONE',  ( -9.431729376590999081, -76.99603667140100072, 1.293989273348000069 ) ) ;
#52595=CARTESIAN_POINT ( 'NONE',  ( -0.6471704932797999188, -78.07045584965399598, 9.701898969124000516 ) ) ;
#52603=CARTESIAN_POINT ( 'NONE',  ( 0.000000000000000000, -75.00000000000000000, -7.200000000000000178 ) ) ;
#52619=CARTESIAN_POINT ( 'NONE',  ( 0.000000000000000000, -75.09999999996229292, 0.000000000000000000 ) ) ;
#52624=CARTESIAN_POINT ( 'NONE',  ( 4.044903269867999640, -79.05999999999998806, -8.595856998426999240 ) ) ;
#52637=CARTESIAN_POINT ( 'NONE',  ( -9.721629130303000466, -78.68311332859899210, 1.228127365514999791 ) ) ;
#52697=EDGE_LOOP ( 'NONE', ( #4964, #36774, #31474, #49512 ) ) ;
#52706=CARTESIAN_POINT ( 'NONE',  ( -2.938756882413333660, -79.29986081116008734, 9.035730373227549350 ) ) ;
#52718=CIRCLE ( 'NONE', #1825, 5.299999999999999822 ) ;
#52726=AXIS2_PLACEMENT_3D ( 'NONE', #30798, #8969, #39956 ) ;
#52727=DIRECTION ( 'NONE',  ( -1.000000000000000000, 0.000000000000000000, 0.000000000000000000 ) ) ;
#52737=CARTESIAN_POINT ( 'NONE',  ( -8.300970689365467337, -78.35833333333332007, 4.784380313523513450 ) ) ;
#52739=CARTESIAN_POINT ( 'NONE',  ( -7.470012560788926947, -78.95333333333331893, -5.923033143556039271 ) ) ;
#52743=DIRECTION ( 'NONE',  ( -0.7071067811865470176, -0.7071067811865470176, -3.647649194621239524E-08 ) ) ;
#52758=EDGE_LOOP ( 'NONE', ( #56380, #48223, #40165, #34671 ) ) ;
#52771=VERTEX_POINT ( 'NONE', #50219 ) ;
#52787=CARTESIAN_POINT ( 'NONE',  ( 9.468102369896000070, -78.02648667140100258, 2.380303120989999854 ) ) ;
#52862=CARTESIAN_POINT ( 'NONE',  ( 9.500000000000003553, -77.04166666666665719, -0.9948376736368218509 ) ) ;
#52880=CARTESIAN_POINT ( 'NONE',  ( -8.871933854994999535, -78.66360194988500609, -3.979018739998999354 ) ) ;
#52898=EDGE_LOOP ( 'NONE', ( #56728, #45821, #12758, #22035 ) ) ;
#52911=SURFACE_STYLE_FILL_AREA ( #12180 ) ;
#52922=CARTESIAN_POINT ( 'NONE',  ( 4.686931394918000038, -78.92108667140098532, -8.732305124302000010 ) ) ;
#52926=VERTEX_POINT ( 'NONE', #44835 ) ;
#52934=EDGE_CURVE ( 'NONE', #34669, #24677, #5056, .T. ) ;
#52935=CARTESIAN_POINT ( 'NONE',  ( -9.308871466119949645, -79.41571124415816030, -1.914396136332924270 ) ) ;
#52975=CARTESIAN_POINT ( 'NONE',  ( 8.150225256662000817, -79.72064415034598994, -4.374508917085999649 ) ) ;
#52995=CARTESIAN_POINT ( 'NONE',  ( 1.305056903442745497, -79.26396365760838592, 9.410159162297995650 ) ) ;
#53065=AXIS2_PLACEMENT_3D ( 'NONE', #47548, #34202, #56381 ) ;
#53075=CARTESIAN_POINT ( 'NONE',  ( 5.982226491729999651, -77.14386001420199079, 7.853930782076001371 ) ) ;
#53095=B_SPLINE_CURVE_WITH_KNOTS ( 'NONE', 3,
 ( #11199, #16197, #42486, #42193, #43346, #33315, #20903, #56925, #11766, #33606, #38906, #24177, #7327, #15321, #55774, #2338, #46932, #47795, #2624, #16484, #1762, #38043, #15902, #51349, #34463, #19756, #52494, #24762, #2055, #6754, #6459, #12051, #46639, #33888, #51929 ),
 .UNSPECIFIED., .F., .F.,
 ( 4, 1, 1, 1, 1, 1, 1, 1, 1, 1, 1, 1, 1, 1, 1, 1, 1, 1, 1, 1, 1, 1, 1, 1, 1, 1, 1, 1, 1, 1, 1, 1, 4 ),
 ( 0.000000000000000000, 0.01250358773558132505, 0.04500335175853042990, 0.07750311578147953129, 0.1100028798044286465, 0.1425026438273777341, 0.1750024078503268354, 0.2075021718732759646, 0.2400019358962250660, 0.2725016999191742229, 0.3050014639421232965, 0.3375012279650724256, 0.3700009919880215548, 0.4025007560109706839, 0.4350005200339197575, 0.4675002840568688867, 0.5000000480798180158, 0.5324998121027670894, 0.5649995761257161631, 0.5974993401486653477, 0.6299991041716144213, 0.6624988681945634950, 0.6949986322175125686, 0.7274983962404617532, 0.7599981602634108269, 0.7924979242863599005, 0.8249976883093089741, 0.8574974523322581588, 0.8899972163552072324, 0.9224969803781563060, 0.9549967444011054907, 0.9874965084240546753, 1.000000000000000000 ),
 .UNSPECIFIED. ) ;
#53111=CARTESIAN_POINT ( 'NONE',  ( -6.786047990210001046, -79.69408667140099567, 6.837407397534001063 ) ) ;
#53118=CARTESIAN_POINT ( 'NONE',  ( -9.252740428349007118, -78.37916666666666288, 2.486604901413125734 ) ) ;
#53130=CARTESIAN_POINT ( 'NONE',  ( 7.430757984336000099, -77.49363084965399651, 5.911115298933000695 ) ) ;
#53163=CARTESIAN_POINT ( 'NONE',  ( 4.294001957131981406, -77.00000000000001421, 8.218741086766758741 ) ) ;
#53166=CARTESIAN_POINT ( 'NONE',  ( -7.530775182571000315, -78.24465584965399501, -6.150709233331999037 ) ) ;
#53181=CYLINDRICAL_SURFACE ( 'NONE', #10732, 11.65000000000000036 ) ;
#53207=CARTESIAN_POINT ( 'NONE',  ( 8.353603324983998490, -78.83708998579800209, -4.904950430745999235 ) ) ;
#53218=CARTESIAN_POINT ( 'NONE',  ( -9.106090911476261596, -79.42266151531977414, -2.710111362998674167 ) ) ;
#53224=CARTESIAN_POINT ( 'NONE',  ( -9.497676279887681261, -79.29010717161661148, 1.243618956522032581 ) ) ;
#53244=CARTESIAN_POINT ( 'NONE',  ( -7.596835002782709623, -77.35208333333333997, -5.838193839761696147 ) ) ;
#53281=CARTESIAN_POINT ( 'NONE',  ( -7.344791241739323517, -79.34486898742505900, 6.031409305879527949 ) ) ;
#53315=CARTESIAN_POINT ( 'NONE',  ( 7.479111157460000214, -79.76976001420199225, -5.552063387031999753 ) ) ;
#53334=AXIS2_PLACEMENT_3D ( 'NONE', #27012, #40007, #26423 ) ;
#53357=DIRECTION ( 'NONE',  ( 0.000000000000000000, 1.000000000000000000, 0.000000000000000000 ) ) ;
#53359=CARTESIAN_POINT ( 'NONE',  ( -9.594333265089000307, -77.77168667140099956, -1.805238218963999941 ) ) ;
#53369=EDGE_CURVE ( 'NONE', #37236, #41372, #4859, .T. ) ;
#53377=VECTOR ( 'NONE', #48320, 1000.000000000000114 ) ;
#53393=CARTESIAN_POINT ( 'NONE',  ( 9.500000000000000000, -78.54999999999999716, 0.000000000000000000 ) ) ;
#53402=ADVANCED_FACE ( 'NONE', ( #12109 ), #22636, .F. ) ;
#53408=ADVANCED_FACE ( 'NONE', ( #38325 ), #29172, .T. ) ;
#53411=DIRECTION ( 'NONE',  ( 0.000000000000000000, -1.000000000000000000, 0.000000000000000000 ) ) ;
#53425=CIRCLE ( 'NONE', #8179, 9.499999999999996447 ) ;
#53439=CARTESIAN_POINT ( 'NONE',  ( -9.539271075714001569, -76.93226332859899230, 1.308743492807000086 ) ) ;
#53452=CARTESIAN_POINT ( 'NONE',  ( -7.401612602209000968, -79.06599415034600042, -6.305503003149000030 ) ) ;
#53495=CARTESIAN_POINT ( 'NONE',  ( -8.838907858698000553, -78.66288998579800307, -3.964206742940000083 ) ) ;
#53505=CARTESIAN_POINT ( 'NONE',  ( -4.784380313523539208, -77.48333333333332007, -8.300970689365453126 ) ) ;
#53509=CARTESIAN_POINT ( 'NONE',  ( -8.578468486503851409, -79.43533626687298010, -4.083052076949801545 ) ) ;
#53510=LINE ( 'NONE', #30189, #2578 ) ;
#53522=DIRECTION ( 'NONE',  ( 0.000000000000000000, -1.000000000000000000, 0.000000000000000000 ) ) ;
#53544=CARTESIAN_POINT ( 'NONE',  ( -6.100000000000000533, -80.79999999999999716, 0.000000000000000000 ) ) ;
#53577=CARTESIAN_POINT ( 'NONE',  ( -7.649979009965352184, -79.34907697906386659, 5.632330841050999126 ) ) ;
#53581=VERTEX_POINT ( 'NONE', #28219 ) ;
#53597=ADVANCED_FACE ( 'NONE', ( #46567 ), #6706, .F. ) ;
#53610=CARTESIAN_POINT ( 'NONE',  ( 6.454959760337000141, -79.25496001420199832, -6.996333296700000481 ) ) ;
#53658=CARTESIAN_POINT ( 'NONE',  ( -4.421234056401999624, -77.84448667140100042, -8.704183203973999028 ) ) ;
#53660=EDGE_CURVE ( 'NONE', #5139, #34611, #16124, .T. ) ;
#53666=CARTESIAN_POINT ( 'NONE',  ( 1.813979036993000227, -79.50980095943377535, 9.381055131006998948 ) ) ;
#53698=CARTESIAN_POINT ( 'NONE',  ( 3.048335112825000248, -79.40808667140099431, -8.921746513659998712 ) ) ;
#53742=CARTESIAN_POINT ( 'NONE',  ( -1.206786224403999963, -77.32811332859900233, 9.552696603499001071 ) ) ;
#53750=CARTESIAN_POINT ( 'NONE',  ( 0.000000000000000000, -75.10000000284179578, -7.200000000000000178 ) ) ;
#53754=CARTESIAN_POINT ( 'NONE',  ( 9.345760913908002010, -78.28209415034599772, 2.683384691900000174 ) ) ;
#53791=CARTESIAN_POINT ( 'NONE',  ( -7.634644595683999668, -77.68053998579799213, -5.724755653662000121 ) ) ;
#53809=CARTESIAN_POINT ( 'NONE',  ( -9.030529600513531818, -79.42482680610650903, -2.948931173546283979 ) ) ;
#53814=CARTESIAN_POINT ( 'NONE',  ( 2.486903332704932801, -79.15440197946847434, 9.251043845573130753 ) ) ;
#53818=AXIS2_PLACEMENT_3D ( 'NONE', #8439, #504, #31740 ) ;
#53839=CARTESIAN_POINT ( 'NONE',  ( -5.838193839761688153, -77.37291666666669698, -7.596835002782716728 ) ) ;
#53857=CARTESIAN_POINT ( 'NONE',  ( -9.500000000000000000, -77.79999999999999716, 0.000000000000000000 ) ) ;
#53878=CARTESIAN_POINT ( 'NONE',  ( -1.291158054771311958, -79.28560666305160964, 9.411828421188701554 ) ) ;
#53895=CYLINDRICAL_SURFACE ( 'NONE', #23725, 1.000000000000000000 ) ;
#53911=AXIS2_PLACEMENT_3D ( 'NONE', #33963, #11837, #29818 ) ;
#53924=ADVANCED_FACE ( 'NONE', ( #50545 ), #14796, .T. ) ;
#53961=CARTESIAN_POINT ( 'NONE',  ( -9.702495711998999184, -77.83546001420199900, -1.825589709539000127 ) ) ;
#53968=CARTESIAN_POINT ( 'NONE',  ( -9.554796630153999715, -79.65020095943376077, -0.02401403847836000235 ) ) ;
#53986=FACE_OUTER_BOUND ( 'NONE', #2395, .T. ) ;
#53995=CARTESIAN_POINT ( 'NONE',  ( 9.397888517861000324, -79.43011332859899198, -1.549072035286999993 ) ) ;
#54005=CIRCLE ( 'NONE', #29503, 1.199999999999999956 ) ;
#54015=CARTESIAN_POINT ( 'NONE',  ( 9.136202122873999798, -77.34189805011500596, 2.585973524422000125 ) ) ;
#54036=CARTESIAN_POINT ( 'NONE',  ( 9.623577716457999642, -77.69568832859899032, 0.3115139696998999730 ) ) ;
#54049=CARTESIAN_POINT ( 'NONE',  ( 9.468750000004000356, -79.53124999999600675, -6.681056941828999630E-10 ) ) ;
#54050=CARTESIAN_POINT ( 'NONE',  ( 7.920136950582000068, -77.80304415034599685, 4.778486233528999705 ) ) ;
#54055=ORIENTED_EDGE ( 'NONE', *, *, #52301, .F. ) ;
#54056=CARTESIAN_POINT ( 'NONE',  ( -4.855043705795097253, -78.21750000000001535, 8.214633846514278304 ) ) ;
#54090=CARTESIAN_POINT ( 'NONE',  ( -0.8449659473473000171, -79.01128998579800111, 9.650246712936999316 ) ) ;
#54101=CARTESIAN_POINT ( 'NONE',  ( -4.778511751969061194, -79.48269898195434280, -8.212683968085311648 ) ) ;
#54119=CARTESIAN_POINT ( 'NONE',  ( -4.784380313523538319, -78.38333333333332575, -8.300970689365453126 ) ) ;
#54125=CARTESIAN_POINT ( 'NONE',  ( -4.802567994450000377, -77.23279903538302449, -8.191018798270000900 ) ) ;
#54129=CARTESIAN_POINT ( 'NONE',  ( 1.243547092045970581, -77.43541666666665435, -9.500000000000000000 ) ) ;
#54145=EDGE_CURVE ( 'NONE', #8940, #41814, #25609, .T. ) ;
#54167=CARTESIAN_POINT ( 'NONE',  ( -9.472578462795231857, -79.39381934248991968, 0.7201139491716196384 ) ) ;
#54204=CARTESIAN_POINT ( 'NONE',  ( -2.309360228211999821, -79.67616001420199723, -9.234877421806000797 ) ) ;
#54254=LINE ( 'NONE', #12417, #48760 ) ;
#54287=CARTESIAN_POINT ( 'NONE',  ( 7.128677745341877703, -78.10833333333332007, 6.432089047655188629 ) ) ;
#54293=CARTESIAN_POINT ( 'NONE',  ( -9.129633152678000130, -79.71611332859899335, -2.714724896223999817 ) ) ;
#54309=DIRECTION ( 'NONE',  ( 0.000000000000000000, 1.000000000000000000, 0.000000000000000000 ) ) ;
#54312=CARTESIAN_POINT ( 'NONE',  ( -2.712012240502000182, -77.46799805011498563, 9.099584490865000319 ) ) ;
#54332=CARTESIAN_POINT ( 'NONE',  ( 8.730183855576999719, -77.15846332859899803, -4.061309546832000628 ) ) ;
#54343=CARTESIAN_POINT ( 'NONE',  ( -7.603664017118000551, -78.51639805011500073, 6.060370778711000384 ) ) ;
#54370=CARTESIAN_POINT ( 'NONE',  ( -1.199999995321999968, -75.00000000467838390, -7.200000027511999079 ) ) ;
#54389=CARTESIAN_POINT ( 'NONE',  ( 8.396442233597756655, -79.33930282387936472, 4.561172822325269216 ) ) ;
#54424=CARTESIAN_POINT ( 'NONE',  ( 2.962511214703000384, -77.80024903538301828, -9.021140561863999707 ) ) ;
#54482=CARTESIAN_POINT ( 'NONE',  ( -9.676327351641999641, -79.01948667140098337, -1.545051445613999874 ) ) ;
#54583=CARTESIAN_POINT ( 'NONE',  ( -9.025535990598001490, -79.65233998579800812, -2.683771280366999523 ) ) ;
#54602=CARTESIAN_POINT ( 'NONE',  ( -7.591316436381999821, -77.12122305011499179, -5.703451837412999659 ) ) ;
#54610=CARTESIAN_POINT ( 'NONE',  ( 5.838193839761673054, -77.62291666666669698, 7.596835002782728274 ) ) ;
#54622=CARTESIAN_POINT ( 'NONE',  ( 9.705941689622999746, -77.12296498579800641, -0.7792165775660999660 ) ) ;
#54652=ADVANCED_FACE ( 'NONE', ( #13722 ), #53895, .F. ) ;
#54653=CARTESIAN_POINT ( 'NONE',  ( -4.681555824253774922, -76.99999999999998579, -8.244243791166322666 ) ) ;
#54659=CARTESIAN_POINT ( 'NONE',  ( -3.781264912327570116, -79.74479166666647245, -8.502894493265863218 ) ) ;
#54683=DIRECTION ( 'NONE',  ( 0.000000000000000000, 1.000000000000000000, 0.000000000000000000 ) ) ;
#54703=CARTESIAN_POINT ( 'NONE',  ( -4.342561293556999935, -77.73719903538301423, -8.443909622126001935 ) ) ;
#54724=CARTESIAN_POINT ( 'NONE',  ( -9.499999999999998224, -77.81041666666665435, -1.243547092045960367 ) ) ;
#54744=B_SPLINE_CURVE_WITH_KNOTS ( 'NONE', 3,
 ( #49713, #4238, #57965, #13964 ),
 .UNSPECIFIED., .F., .F.,
 ( 4, 4 ),
 ( 0.000000000000000000, 1.000000000000000000 ),
 .UNSPECIFIED. ) ;
#54745=ORIENTED_EDGE ( 'NONE', *, *, #21135, .F. ) ;
#54747=DIRECTION ( 'NONE',  ( 0.000000000000000000, 1.000000000000000000, 0.000000000000000000 ) ) ;
#54757=CARTESIAN_POINT ( 'NONE',  ( -7.731096697273209806, -77.00347157156862465, 5.096092861886030612 ) ) ;
#54762=CARTESIAN_POINT ( 'NONE',  ( 2.006136628026000235, -78.21226001420198770, -9.477164255927000625 ) ) ;
#54794=CARTESIAN_POINT ( 'NONE',  ( 0.000000000000000000, -75.00000000000000000, 7.200000000000000178 ) ) ;
#54827=CARTESIAN_POINT ( 'NONE',  ( -8.296701268784000050, -77.03153501420199234, 4.443109075551999965 ) ) ;
#54832=CARTESIAN_POINT ( 'NONE',  ( 1.856358691897999957, -77.05271332859899758, 9.472443054301999510 ) ) ;
#54880=CARTESIAN_POINT ( 'NONE',  ( 8.979348251287998295, -77.84629805011500991, 3.086914251890999772 ) ) ;
#54934=CARTESIAN_POINT ( 'NONE',  ( -9.295554138914937425, -76.99999999999998579, -1.018217055612035127 ) ) ;
#54944=CARTESIAN_POINT ( 'NONE',  ( 8.072669757012000957, -77.73631332859899601, 4.870514429535999668 ) ) ;
#54972=EDGE_CURVE ( 'NONE', #53581, #29780, #34914, .T. ) ;
#54974=VERTEX_POINT ( 'NONE', #52624 ) ;
#54990=ORIENTED_EDGE ( 'NONE', *, *, #24918, .T. ) ;
#54991=CARTESIAN_POINT ( 'NONE',  ( -9.061228178001998756, -77.67414903538301019, -2.837532765875999896 ) ) ;
#55002=CYLINDRICAL_SURFACE ( 'NONE', #11316, 9.500000000000000000 ) ;
#55031=CARTESIAN_POINT ( 'NONE',  ( -9.943323471430000282, -78.81066001420198575, 1.256133873833999992 ) ) ;
#55034=ORIENTED_EDGE ( 'NONE', *, *, #6635, .T. ) ;
#55069=CARTESIAN_POINT ( 'NONE',  ( 0.000000000000000000, -78.00000000000000000, 7.200000000000000178 ) ) ;
#55079=FACE_OUTER_BOUND ( 'NONE', #17454, .T. ) ;
#55080=CARTESIAN_POINT ( 'NONE',  ( 0.000000000000000000, -80.70000000003399521, 0.000000000000000000 ) ) ;
#55083=CARTESIAN_POINT ( 'NONE',  ( 5.838193839761669501, -77.22291666666666288, 7.596835002782726498 ) ) ;
#55086=EDGE_CURVE ( 'NONE', #40996, #15146, #9491, .T. ) ;
#55098=CARTESIAN_POINT ( 'NONE',  ( 9.500000000000000000, -79.14999999999999147, 0.000000000000000000 ) ) ;
#55103=DIRECTION ( 'NONE',  ( 0.000000000000000000, 1.000000000000000000, 0.000000000000000000 ) ) ;
#55114=CARTESIAN_POINT ( 'NONE',  ( -4.747522457205999302, -77.65358501420199389, -8.126364432035000362 ) ) ;
#55122=CARTESIAN_POINT ( 'NONE',  ( 8.125826840328944201, -77.10625000000000284, -4.977714890814727511 ) ) ;
#55132=CARTESIAN_POINT ( 'NONE',  ( -9.500000000000000000, -77.89999999999999147, 0.000000000000000000 ) ) ;
#55176=CARTESIAN_POINT ( 'NONE',  ( 4.001451577097999923, -77.90934805011499975, 8.339717337904000161 ) ) ;
#55192=CYLINDRICAL_SURFACE ( 'NONE', #25161, 9.199999999999999289 ) ;
#55196=AXIS2_PLACEMENT_3D ( 'NONE', #23467, #42365, #28174 ) ;
#55226=CARTESIAN_POINT ( 'NONE',  ( -5.638272052137092594, -76.99999999999998579, -7.602424392853662560 ) ) ;
#55237=CARTESIAN_POINT ( 'NONE',  ( 2.078959492154019095, -77.75750000000002160, 9.312872062229846648 ) ) ;
#55250=CARTESIAN_POINT ( 'NONE',  ( 0.000000000000000000, -74.70999999999999375, 0.000000000000000000 ) ) ;
#55281=CARTESIAN_POINT ( 'NONE',  ( -7.264520526674997924, -77.70567403538302642, -6.114261184555999762 ) ) ;
#55305=CARTESIAN_POINT ( 'NONE',  ( 4.784380313523556083, -77.96666666666666856, -8.300970689365444244 ) ) ;
#55316=ORIENTED_EDGE ( 'NONE', *, *, #16724, .T. ) ;
#55322=CARTESIAN_POINT ( 'NONE',  ( -7.837473280028000033, -78.76711001420200375, 6.246724465767999668 ) ) ;
#55339=CARTESIAN_POINT ( 'NONE',  ( -7.931488639841374422, -77.09554693750341414, -5.131895770657950884 ) ) ;
#55344=CARTESIAN_POINT ( 'NONE',  ( 6.458817137649000450, -79.25746001420199605, -6.573457973844999636 ) ) ;
#55351=CARTESIAN_POINT ( 'NONE',  ( 0.000000000000000000, -74.70999999999999375, 0.000000000000000000 ) ) ;
#55371=CARTESIAN_POINT ( 'NONE',  ( -8.630067035710000667, -79.60524805011499438, -4.100810385846999750 ) ) ;
#55375=CARTESIAN_POINT ( 'NONE',  ( -8.300970689365467337, -77.35833333333330586, 4.784380313523513450 ) ) ;
#55383=CIRCLE ( 'NONE', #44050, 1.000000000000000000 ) ;
#55408=CARTESIAN_POINT ( 'NONE',  ( -8.899304630592000720, -77.59703501420199245, -3.062539053741000217 ) ) ;
#55426=CARTESIAN_POINT ( 'NONE',  ( 4.598371993787000456, -78.67404415034599197, -8.567308531191999421 ) ) ;
#55464=EDGE_LOOP ( 'NONE', ( #48356, #34536, #12538 ) ) ;
#55466=DIRECTION ( 'NONE',  ( -1.000000000000000000, 0.000000000000000000, 0.000000000000000000 ) ) ;
#55469=CARTESIAN_POINT ( 'NONE',  ( -2.712012240502000182, -77.40789415034599585, 9.099584490865000319 ) ) ;
#55488=CARTESIAN_POINT ( 'NONE',  ( -8.583774432395999909, -76.84021498579799925, 4.596844558760999178 ) ) ;
#55531=CARTESIAN_POINT ( 'NONE',  ( -7.629208874607999569, -78.93548998579800013, -6.499394396314999156 ) ) ;
#55556=CARTESIAN_POINT ( 'NONE',  ( 5.836375128730250772, -79.12308539666503293, 7.594790468097947667 ) ) ;
#55568=LINE ( 'NONE', #15418, #27364 ) ;
#55599=B_SPLINE_CURVE_WITH_KNOTS ( 'NONE', 3,
 ( #26850, #9158, #12977, #12416, #52862, #57863 ),
 .UNSPECIFIED., .F., .F.,
 ( 4, 2, 4 ),
 ( 0.000000000000000000, 0.5000000000000000000, 1.000000000000000000 ),
 .UNSPECIFIED. ) ;
#55615=PRODUCT_CONTEXT ( 'NONE', #48140, 'mechanical' ) ;
#55636=CARTESIAN_POINT ( 'NONE',  ( -0.6447613848864999220, -77.95096001420199627, 9.665783406873000416 ) ) ;
#55642=CARTESIAN_POINT ( 'NONE',  ( 0.000000000000000000, -74.70999999999999375, 0.000000000000000000 ) ) ;
#55656=CARTESIAN_POINT ( 'NONE',  ( 9.129467682721999822, -79.09873998579800514, -3.694451172265999617 ) ) ;
#55661=CARTESIAN_POINT ( 'NONE',  ( -8.871933854994999535, -78.68354514476064310, -3.979018739998999354 ) ) ;
#55665=DIRECTION ( 'NONE',  ( 0.000000000000000000, 0.000000000000000000, -1.000000000000000000 ) ) ;
#55669=CARTESIAN_POINT ( 'NONE',  ( 2.905710065331635228, -79.62500000110051701, -8.943793168028266294 ) ) ;
#55687=CARTESIAN_POINT ( 'NONE',  ( 7.735842139137476536, -79.19900585853359587, 5.514108658314483158 ) ) ;
#55706=CARTESIAN_POINT ( 'NONE',  ( -6.984884556549999957, -77.51221001420199741, 6.307785355753999568 ) ) ;
#55709=CARTESIAN_POINT ( 'NONE',  ( 0.000000000000000000, -80.79999999999999716, 0.000000000000000000 ) ) ;
#55723=CONICAL_SURFACE ( 'NONE', #40628, 1.099999997158000120, 0.7853981633972997312 ) ;
#55759=ORIENTED_EDGE ( 'NONE', *, *, #28870, .T. ) ;
#55770=CARTESIAN_POINT ( 'NONE',  ( 7.430757984336000099, -77.31331915034598978, 5.911115298933000695 ) ) ;
#55774=CARTESIAN_POINT ( 'NONE',  ( -0.5313338453197881117, -78.66977913613844464, -9.710363398104801647 ) ) ;
#55793=DIRECTION ( 'NONE',  ( -1.000000000000000000, 0.000000000000000000, 0.000000000000000000 ) ) ;
#55821=CARTESIAN_POINT ( 'NONE',  ( -9.098835018745974779, -77.00000000000000000, -2.252957314591238269 ) ) ;
#55830=CARTESIAN_POINT ( 'NONE',  ( -8.500869906239362450, -77.86249999999999716, 4.334382246026820873 ) ) ;
#55834=CARTESIAN_POINT ( 'NONE',  ( -9.128193891305592444, -79.37730585991548082, 2.631818823965640597 ) ) ;
#55837=CYLINDRICAL_SURFACE ( 'NONE', #47649, 11.65000000000000036 ) ;
#55885=DIRECTION ( 'NONE',  ( -1.044282756598000039E-09, -1.000000000000000000, 6.141137129051000072E-09 ) ) ;
#55896=CARTESIAN_POINT ( 'NONE',  ( 7.596835002782722057, -77.99791666666666856, -5.838193839761678383 ) ) ;
#55901=CIRCLE ( 'NONE', #29492, 1.000000000000000000 ) ;
#55911=CIRCLE ( 'NONE', #53065, 6.100000000000000533 ) ;
#55916=CARTESIAN_POINT ( 'NONE',  ( -5.941820572504999731, -79.24616001420199041, 8.071079272148001138 ) ) ;
#55934=VECTOR ( 'NONE', #21282, 1000.000000000000227 ) ;
#55935=CARTESIAN_POINT ( 'NONE',  ( -5.548464554217999556, -78.58398667140099292, -8.076689350464999251 ) ) ;
#55940=FACE_OUTER_BOUND ( 'NONE', #3047, .T. ) ;
#55942=CARTESIAN_POINT ( 'NONE',  ( 0.000000000000000000, -75.10000000284179578, 7.200000000000000178 ) ) ;
#55954=CARTESIAN_POINT ( 'NONE',  ( 2.854995274860000265, -79.02853998579799111, -9.096945719287999665 ) ) ;
#55961=CARTESIAN_POINT ( 'NONE',  ( 8.150225256662000817, -79.84085194988499268, -4.374508917085999649 ) ) ;
#55972=ORIENTED_EDGE ( 'NONE', *, *, #42483, .F. ) ;
#55981=CARTESIAN_POINT ( 'NONE',  ( 6.183015154944156322, -79.21846095476607275, 7.212400455461417614 ) ) ;
#56003=CARTESIAN_POINT ( 'NONE',  ( 5.838193839761673054, -77.12291666666669698, 7.596835002782728274 ) ) ;
#56013=VECTOR ( 'NONE', #36513, 1000.000000000000000 ) ;
#56035=ORIENTED_EDGE ( 'NONE', *, *, #56145, .F. ) ;
#56065=DIRECTION ( 'NONE',  ( 0.000000000000000000, 1.000000000000000000, 0.000000000000000000 ) ) ;
#56124=CARTESIAN_POINT ( 'NONE',  ( -9.470785009285748401, -79.39361871371332313, 0.7431805272417587593 ) ) ;
#56126=DIRECTION ( 'NONE',  ( 0.000000000000000000, -1.000000000000000000, 0.000000000000000000 ) ) ;
#56145=EDGE_CURVE ( 'NONE', #39734, #40288, #37868, .T. ) ;
#56204=CARTESIAN_POINT ( 'NONE',  ( -5.611728806388999402, -78.83398667140099292, -8.168780722191000265 ) ) ;
#56222=CARTESIAN_POINT ( 'NONE',  ( -7.544159220956999867, -78.99926332859899958, -6.426939800899999611 ) ) ;
#56246=FACE_BOUND ( 'NONE', #5280, .T. ) ;
#56250=CARTESIAN_POINT ( 'NONE',  ( 9.345760913908002010, -78.42224514476065167, 2.683384691899999730 ) ) ;
#56253=CARTESIAN_POINT ( 'NONE',  ( 1.813979036992999783, -79.48985194988500780, 9.381055131006998948 ) ) ;
#56257=CARTESIAN_POINT ( 'NONE',  ( 6.582919022827243616, -79.71875000027529268, -6.583307224015771730 ) ) ;
#56271=CARTESIAN_POINT ( 'NONE',  ( 7.654057555294024873, -79.20013708438366962, 5.626991512746083224 ) ) ;
#56275=ORIENTED_EDGE ( 'NONE', *, *, #39148, .T. ) ;
#56291=CARTESIAN_POINT ( 'NONE',  ( 9.252740428348991131, -77.07083333333333997, 2.486604901413179913 ) ) ;
#56311=VERTEX_POINT ( 'NONE', #6700 ) ;
#56324=DIRECTION ( 'NONE',  ( -0.7071067811865470176, -0.7071067811865470176, -3.647648880603240205E-08 ) ) ;
#56345=CARTESIAN_POINT ( 'NONE',  ( 2.962511214703000384, -77.66009415034599783, -9.021140561863999707 ) ) ;
#56359=CARTESIAN_POINT ( 'NONE',  ( -1.243547092045951263, -78.01458333333333428, -9.500000000000003553 ) ) ;
#56369=ADVANCED_FACE ( 'NONE', ( #11148 ), #46876, .T. ) ;
#56380=ORIENTED_EDGE ( 'NONE', *, *, #821, .F. ) ;
#56381=DIRECTION ( 'NONE',  ( -1.000000000000000000, 0.000000000000000000, 0.000000000000000000 ) ) ;
#56395=CARTESIAN_POINT ( 'NONE',  ( 0.000000000000000000, -76.00000000000000000, 0.000000000000000000 ) ) ;
#56400=AXIS2_PLACEMENT_3D ( 'NONE', #14053, #32048, #6070 ) ;
#56415=EDGE_CURVE ( 'NONE', #14353, #13828, #55568, .T. ) ;
#56420=EDGE_LOOP ( 'NONE', ( #19320, #32336, #17441, #12535 ) ) ;
#56460=ADVANCED_FACE ( 'NONE', ( #2146 ), #48868, .F. ) ;
#56492=CARTESIAN_POINT ( 'NONE',  ( -3.365558374102000094, -78.59601332859899969, 9.202792326454000360 ) ) ;
#56509=CARTESIAN_POINT ( 'NONE',  ( -3.292576784871000140, -78.04116332859899785, -9.347695904456999827 ) ) ;
#56516=CARTESIAN_POINT ( 'NONE',  ( 9.500000000000000000, -78.14999999999999147, 0.000000000000000000 ) ) ;
#56536=CARTESIAN_POINT ( 'NONE',  ( -3.339615680725999791, -78.55289514476064028, 9.131854552393999569 ) ) ;
#56556=CARTESIAN_POINT ( 'NONE',  ( 7.901592333655654166, -79.19663653965405103, 5.277476999614962416 ) ) ;
#56581=DIRECTION ( 'NONE',  ( 0.000000000000000000, 1.000000000000000000, 0.000000000000000000 ) ) ;
#56587=CARTESIAN_POINT ( 'NONE',  ( 0.000000000000000000, -75.09999999996229292, 0.000000000000000000 ) ) ;
#56596=CARTESIAN_POINT ( 'NONE',  ( 1.199999995321999968, -75.00000000467838390, -7.199999972488000388 ) ) ;
#56621=ORIENTED_EDGE ( 'NONE', *, *, #49946, .F. ) ;
#56640=EDGE_CURVE ( 'NONE', #54974, #16476, #9010, .T. ) ;
#56647=CARTESIAN_POINT ( 'NONE',  ( 9.574841743191999655, -78.09026001420200203, 2.407137649543000357 ) ) ;
#56652=CARTESIAN_POINT ( 'NONE',  ( 9.199999999999999289, -77.00000000000000000, 0.000000000000000000 ) ) ;
#56717=UNCERTAINTY_MEASURE_WITH_UNIT (LENGTH_MEASURE( 1.000000000000000082E-05 ), #47884, 'distance_accuracy_value', 'NONE');
#56726=LINE ( 'NONE', #19841, #47025 ) ;
#56728=ORIENTED_EDGE ( 'NONE', *, *, #17154, .F. ) ;
#56738=CARTESIAN_POINT ( 'NONE',  ( 2.013632425233999879, -78.27165194988499763, -9.512575055159999238 ) ) ;
#56779=CARTESIAN_POINT ( 'NONE',  ( 4.634092916811999530, -78.85731332859899112, -8.633860817301998836 ) ) ;
#56780=DIRECTION ( 'NONE',  ( 0.000000000000000000, 0.000000000000000000, -1.000000000000000000 ) ) ;
#56791=LINE ( 'NONE', #20202, #40750 ) ;
#56798=CARTESIAN_POINT ( 'NONE',  ( 2.029274658824999911, -78.14848667140098826, -9.586470329786999756 ) ) ;
#56818=CARTESIAN_POINT ( 'NONE',  ( 9.500000000000000000, -79.04999999999999716, 0.000000000000000000 ) ) ;
#56824=DIRECTION ( 'NONE',  ( 0.000000000000000000, -1.000000000000000000, 0.000000000000000000 ) ) ;
#56843=ORIENTED_EDGE ( 'NONE', *, *, #30277, .T. ) ;
#56847=CARTESIAN_POINT ( 'NONE',  ( 2.963863982283218679, -79.24946267513759324, 9.025665246861352742 ) ) ;
#56852=CARTESIAN_POINT ( 'NONE',  ( -8.630529134780177358, -79.58500282387936409, -4.101029964751555568 ) ) ;
#56865=CARTESIAN_POINT ( 'NONE',  ( -7.065445606947000634, -77.44843667140099797, 6.380536996790000082 ) ) ;
#56881=DIRECTION ( 'NONE',  ( 0.000000000000000000, -1.000000000000000000, 0.000000000000000000 ) ) ;
#56906=AXIS2_PLACEMENT_3D ( 'NONE', #5808, #50121, #42130 ) ;
#56925=CARTESIAN_POINT ( 'NONE',  ( -5.765467378296696310, -78.97462913613841806, 7.831529694205842773 ) ) ;
#56963=CARTESIAN_POINT ( 'NONE',  ( -5.141276782405999946, -79.83708667140099635, -8.146626593840000652 ) ) ;
#56980=CARTESIAN_POINT ( 'NONE',  ( 2.459440699436000077, -77.33600584965400060, -9.171074077620000153 ) ) ;
#57003=CARTESIAN_POINT ( 'NONE',  ( -8.392392323321001157, -76.96776167140099290, 4.494354236621999732 ) ) ;
#57013=CARTESIAN_POINT ( 'NONE',  ( 4.495149389856036848, -77.00000000000000000, 8.113504219799731132 ) ) ;
#57016=CARTESIAN_POINT ( 'NONE',  ( -5.600962501326000265, -78.05390194988500241, 7.948110234177999445 ) ) ;
#57052=LINE ( 'NONE', #12459, #9194 ) ;
#57063=CARTESIAN_POINT ( 'NONE',  ( 6.797895215277000247, -78.44203667140099867, -7.211733462747999646 ) ) ;
#57067=ORIENTED_EDGE ( 'NONE', *, *, #51935, .F. ) ;
#57123=VERTEX_POINT ( 'NONE', #1299 ) ;
#57129=CARTESIAN_POINT ( 'NONE',  ( -6.642891787447657848, -79.33646197186951099, 6.791764226237924973 ) ) ;
#57158=DIRECTION ( 'NONE',  ( 0.000000000000000000, 0.000000000000000000, -1.000000000000000000 ) ) ;
#57160=CARTESIAN_POINT ( 'NONE',  ( -9.500000000000000000, -78.89999999999999147, 0.000000000000000000 ) ) ;
#57172=CARTESIAN_POINT ( 'NONE',  ( 0.000000000000000000, -75.20000000000000284, 0.000000000000000000 ) ) ;
#57174=ADVANCED_FACE ( 'NONE', ( #25738 ), #18912, .T. ) ;
#57184=ORIENTED_EDGE ( 'NONE', *, *, #25470, .F. ) ;
#57267=ORIENTED_EDGE ( 'NONE', *, *, #12027, .F. ) ;
#57268=CARTESIAN_POINT ( 'NONE',  ( -4.802567994450000377, -77.27295584965399655, -8.191018798270000900 ) ) ;
#57292=CARTESIAN_POINT ( 'NONE',  ( 4.290841056834999279, -77.78051332859898537, 8.395152818089000490 ) ) ;
#57306=CARTESIAN_POINT ( 'NONE',  ( -9.601739433208001273, -79.14265194988499275, -1.533141744029000053 ) ) ;
#57326=CIRCLE ( 'NONE', #39413, 9.499999999999996447 ) ;
#57343=ORIENTED_EDGE ( 'NONE', *, *, #3507, .F. ) ;
#57348=CARTESIAN_POINT ( 'NONE',  ( 9.525749612248999298, -78.52913667140100529, 2.735063621234999687 ) ) ;
#57369=ORIENTED_EDGE ( 'NONE', *, *, #7385, .F. ) ;
#57385=B_SPLINE_CURVE_WITH_KNOTS ( 'NONE', 3,
 ( #10618, #28600, #29749, #15618, #7623, #21196, #38336, #3206, #2061, #56359, #33613, #7052, #43352, #20062, #15910, #2346, #38629, #51656 ),
 .UNSPECIFIED., .F., .F.,
 ( 4, 2, 2, 2, 2, 2, 2, 2, 4 ),
 ( 0.000000000000000000, 0.1249999999999999445, 0.2499999999999998890, 0.3749999999999998335, 0.4999999999999997780, 0.6249999999999997780, 0.7499999999999997780, 0.8749999999999997780, 1.000000000000000000 ),
 .UNSPECIFIED. ) ;
#57403=CARTESIAN_POINT ( 'NONE',  ( -2.364557222828000072, -79.40474415034600497, 9.257622954664000758 ) ) ;
#57420=CARTESIAN_POINT ( 'NONE',  ( -3.960513469484321813, -79.30881237240771497, 8.637712416346211342 ) ) ;
#57452=CARTESIAN_POINT ( 'NONE',  ( -5.762329935654880941, -78.97333333333331495, -7.594666746517801492 ) ) ;
#57489=CARTESIAN_POINT ( 'NONE',  ( -4.716969250163658423, -79.63541666666263552, 8.182319322371521153 ) ) ;
#57498=CARTESIAN_POINT ( 'NONE',  ( -9.741854131801998662, -77.26208667140099351, -0.6374903164020000457 ) ) ;
#57550=CARTESIAN_POINT ( 'NONE',  ( -5.597970637881999778, -77.11533084965400064, 7.669424558767000022 ) ) ;
#57587=CARTESIAN_POINT ( 'NONE',  ( -3.230363664242999810, -78.28820584965400542, -9.171071524558000121 ) ) ;
#57617=SHAPE_REPRESENTATION_RELATIONSHIP ( 'NONE' , 'NONE' ,  #1422, #1805 ) ;
#57624=CARTESIAN_POINT ( 'NONE',  ( 8.638761211478000135, -76.97991332859899671, 4.306371860147999442 ) ) ;
#57631=CARTESIAN_POINT ( 'NONE',  ( -7.502741683071000089, -78.18383998579800220, -6.127813063941999872 ) ) ;
#57634=ORIENTED_EDGE ( 'NONE', *, *, #3038, .F. ) ;
#57643=CARTESIAN_POINT ( 'NONE',  ( -3.507835537823156713, -79.49465701644101046, -8.848935139560099472 ) ) ;
#57658=CARTESIAN_POINT ( 'NONE',  ( 7.596835002782722057, -78.49791666666666856, -5.838193839761678383 ) ) ;
#57669=CARTESIAN_POINT ( 'NONE',  ( -8.300970689365446020, -77.34166666666666856, -4.784380313523547201 ) ) ;
#57672=CARTESIAN_POINT ( 'NONE',  ( 4.855043705795149656, -79.06749999999999545, -8.214633846514242776 ) ) ;
#57674=CARTESIAN_POINT ( 'NONE',  ( -11.44999999999999929, -75.00000000000000000, 0.000000000000000000 ) ) ;
#57705=CARTESIAN_POINT ( 'NONE',  ( -7.140373151351809611, -79.34225595484394944, 6.275840911652932341 ) ) ;
#57720=CARTESIAN_POINT ( 'NONE',  ( 6.695659669993999863, -77.19396167140099863, -6.767563488957999418 ) ) ;
#57735=CARTESIAN_POINT ( 'NONE',  ( -8.708326823944164019, -78.93333333333330870, -3.879233584792522116 ) ) ;
#57789=CARTESIAN_POINT ( 'NONE',  ( 1.877525114294000153, -77.11648667140100599, 9.580448975616000951 ) ) ;
#57795=CARTESIAN_POINT ( 'NONE',  ( -6.090475762158000350, -79.58000095943376095, 7.362120511650999788 ) ) ;
#57828=ORIENTED_EDGE ( 'NONE', *, *, #6097, .T. ) ;
#57841=EDGE_LOOP ( 'NONE', ( #14922, #17627, #57343, #56035, #14933, #3876, #57267 ) ) ;
#57842=CARTESIAN_POINT ( 'NONE',  ( -7.591316436381999821, -77.24143084965399453, -5.703451837412999659 ) ) ;
#57860=EDGE_CURVE ( 'NONE', #42268, #13828, #14216, .T. ) ;
#57863=CARTESIAN_POINT ( 'NONE',  ( 9.500000000000000000, -77.04999999999999716, 0.000000000000000000 ) ) ;
#57868=CARTESIAN_POINT ( 'NONE',  ( -9.734394856890000725, -77.37743998579799154, 0.2324636006574999636 ) ) ;
#57880=CARTESIAN_POINT ( 'NONE',  ( -5.764562846862999912, -79.05555194988498613, 7.830301022820999712 ) ) ;
#57886=CARTESIAN_POINT ( 'NONE',  ( 2.078959492154019983, -78.15749999999999886, 9.312872062229846648 ) ) ;
#57915=CARTESIAN_POINT ( 'NONE',  ( 7.488372721267999133, -77.82613998579800807, -5.914808301684000291 ) ) ;
#57933=CARTESIAN_POINT ( 'NONE',  ( -7.596835002782708735, -77.45208333333332007, -5.838193839761694370 ) ) ;
#57935=CARTESIAN_POINT ( 'NONE',  ( -9.242397610492675497, -79.41824321304214607, -2.209549243808804686 ) ) ;
#57965=CARTESIAN_POINT ( 'NONE',  ( 6.002063118397120256, -77.76911124895428884, 7.255260483856941889 ) ) ;
#57985=CARTESIAN_POINT ( 'NONE',  ( 0.000000000000000000, -76.00000000000000000, 0.000000000000000000 ) ) ;
#57988=EDGE_LOOP ( 'NONE', ( #51079, #7397, #17848, #58222 ) ) ;
#58000=CARTESIAN_POINT ( 'NONE',  ( 1.487313896732463725, -79.26245606279938727, 9.382830533248572635 ) ) ;
#58012=EDGE_CURVE ( 'NONE', #52771, #40996, #50679, .T. ) ;
#58032=CARTESIAN_POINT ( 'NONE',  ( 2.561895579250705435, -79.04666666666665265, -9.182597689054190937 ) ) ;
#58034=CARTESIAN_POINT ( 'NONE',  ( 5.624272343092999726, -79.39536001420199796, 7.680093418580999476 ) ) ;
#58050=CARTESIAN_POINT ( 'NONE',  ( 0.000000000000000000, -77.00000000000000000, 0.000000000000000000 ) ) ;
#58056=CIRCLE ( 'NONE', #55196, 9.199999999999999289 ) ;
#58082=CARTESIAN_POINT ( 'NONE',  ( -3.703509300394999926, -77.72626001420199771, 9.151787782534000826 ) ) ;
#58089=CARTESIAN_POINT ( 'NONE',  ( 5.645287065787000458, -79.47470095943376123, 7.708789581145001790 ) ) ;
#58126=EDGE_CURVE ( 'NONE', #15737, #8049, #30729, .T. ) ;
#58150=DIRECTION ( 'NONE',  ( -0.7071067811865474617, -0.7071067811865474617, -3.646389762765242273E-10 ) ) ;
#58159=CARTESIAN_POINT ( 'NONE',  ( 5.376571573888999644, -77.20778998579800145, 8.118187030778999613 ) ) ;
#58173=CARTESIAN_POINT ( 'NONE',  ( 2.013632425233999879, -78.21154805011499889, -9.512575055159999238 ) ) ;
#58180=CARTESIAN_POINT ( 'NONE',  ( 0.3023719455682365442, -78.17250000000001364, 9.537307262745171599 ) ) ;
#58203=DIRECTION ( 'NONE',  ( 0.7071067811865470176, -0.7071067811865470176, 3.647649194621239524E-08 ) ) ;
#58213=EDGE_LOOP ( 'NONE', ( #15082, #55759, #24572, #52531, #30288 ) ) ;
#58217=CARTESIAN_POINT ( 'NONE',  ( 7.103190263045000563, -78.00082999526600247, 6.271635551916999951 ) ) ;
#58222=ORIENTED_EDGE ( 'NONE', *, *, #54972, .F. ) ;
#58229=CARTESIAN_POINT ( 'NONE',  ( -7.065921977188095227, -79.45798876533616806, -6.351589347257088569 ) ) ;
#58235=CARTESIAN_POINT ( 'NONE',  ( 1.243096656778429177, -79.16484084040288849, 9.498104304983947088 ) ) ;
#58236=EDGE_CURVE ( 'NONE', #8584, #47685, #25600, .T. ) ;
#58293=AXIS2_PLACEMENT_3D ( 'NONE', #36849, #41578, #9122 ) ;
#58298=CARTESIAN_POINT ( 'NONE',  ( -3.585728412114033148, -79.30548461880201216, 8.797105590405882580 ) ) ;
#58313=CARTESIAN_POINT ( 'NONE',  ( 7.355956161948723704, -77.74587193750340930, -5.927457667800279495 ) ) ;
#58315=CARTESIAN_POINT ( 'NONE',  ( 9.161831023485000003, -77.27878667140099367, 2.587011072425999814 ) ) ;
#58333=CARTESIAN_POINT ( 'NONE',  ( 8.925918906643000028, -79.22628667140099878, -3.612080431657000101 ) ) ;
#58339=CARTESIAN_POINT ( 'NONE',  ( -1.000000000000000000, -78.00000000000000000, -7.200000000000000178 ) ) ;
#58351=ADVANCED_FACE ( 'NONE', ( #21960 ), #18997, .T. ) ;
#58365=ORIENTED_EDGE ( 'NONE', *, *, #32682, .T. ) ;
#58379=CARTESIAN_POINT ( 'NONE',  ( 9.794900829080001259, -77.58066001420199598, 1.237383733679000120 ) ) ;
ENDSEC;
END-ISO-10303-21;
